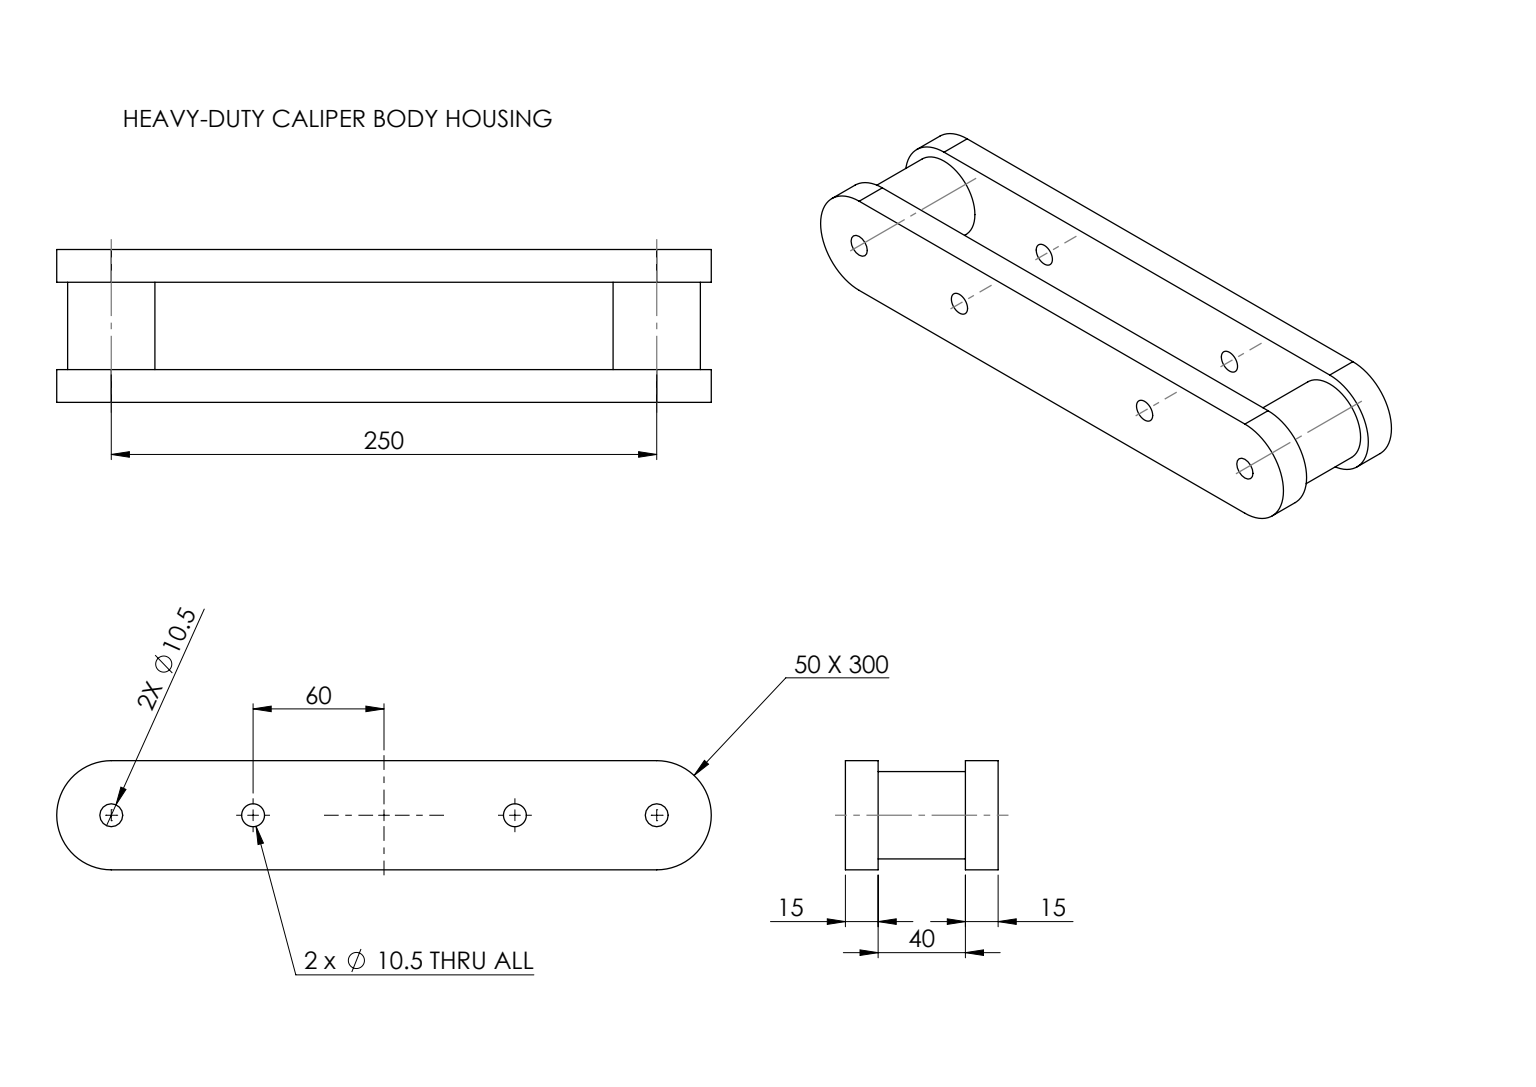
ISO-10303-21;
HEADER;
FILE_DESCRIPTION (('STEP AP214'),
    '1' );
FILE_NAME ('Heavy-Duty Caliper Body Housing.step',
    '2026-10-08T07:58:12',
    ( '' ),
    ( '' ),
    'SwSTEP 2.0',
    'SolidWorks 2026',
    '' );
FILE_SCHEMA (( 'AUTOMOTIVE_DESIGN' ));
ENDSEC;

DATA;
#32=DIRECTION ( 'NONE',  ( -0.000000000000000000, -0.000000000000000000, -1.000000000000000000 ) ) ;
#36=EDGE_CURVE ( 'NONE', #1409, #6493, #16652, .T. ) ;
#53=CARTESIAN_POINT ( 'NONE',  ( 124.3127766070272315, 5.250000000000032863, 35.00001199999999812 ) ) ;
#166=CYLINDRICAL_SURFACE ( 'NONE', #13806, 5.249999999999991118 ) ;
#182=AXIS2_PLACEMENT_3D ( 'NONE', #23295, #23628, #33351 ) ;
#218=CARTESIAN_POINT ( 'NONE',  ( 127.6439996469472220, 4.587378538859885779, 35.00001200000000523 ) ) ;
#239=EDGE_LOOP ( 'NONE', ( #2645, #22396, #19117, #16780 ) ) ;
#303=CARTESIAN_POINT ( 'NONE',  ( 120.4126214611401195, -2.643999646947191362, 35.00001199999999812 ) ) ;
#334=( NAMED_UNIT ( * ) PLANE_ANGLE_UNIT ( ) SI_UNIT ( $, .RADIAN. ) );
#365=ORIENTED_EDGE ( 'NONE', *, *, #11822, .F. ) ;
#449=EDGE_LOOP ( 'NONE', ( #2882, #4117, #25704, #19508 ) ) ;
#451=ORIENTED_EDGE ( 'NONE', *, *, #3089, .T. ) ;
#458=DIRECTION ( 'NONE',  ( 0.000000000000000000, 0.000000000000000000, 1.000000000000000000 ) ) ;
#474=CARTESIAN_POINT ( 'NONE',  ( 122.3560003530528064, -4.587378538859826271, 35.00001200000000523 ) ) ;
#498=CARTESIAN_POINT ( 'NONE',  ( -105.0000000000000142, 2.449293598294705330E-15, 35.00200000000000244 ) ) ;
#553=CARTESIAN_POINT ( 'NONE',  ( -65.24999999999998579, -6.704941225331758039E-15, -20.00000000000000355 ) ) ;
#676=DIRECTION ( 'NONE',  ( -0.000000000000000000, -0.000000000000000000, -1.000000000000000000 ) ) ;
#709=CARTESIAN_POINT ( 'NONE',  ( -125.0000000000000000, 0.000000000000000000, 35.00000000000000000 ) ) ;
#766=PLANE ( 'NONE',  #3114 ) ;
#791=ADVANCED_FACE ( 'NONE', ( #31825 ), #29110, .T. ) ;
#806=CARTESIAN_POINT ( 'NONE',  ( -130.2500000000000000, 6.429395695523609083E-16, 35.00000599999999906 ) ) ;
#827=EDGE_CURVE ( 'NONE', #18269, #18960, #27386, .T. ) ;
#830=EDGE_LOOP ( 'NONE', ( #26379, #19429, #20513, #9975 ) ) ;
#901=AXIS2_PLACEMENT_3D ( 'NONE', #15694, #7192, #17748 ) ;
#981=AXIS2_PLACEMENT_3D ( 'NONE', #30181, #6671, #17224 ) ;
#995=AXIS2_PLACEMENT_3D ( 'NONE', #7458, #17673, #4722 ) ;
#998=ORIENTED_EDGE ( 'NONE', *, *, #28348, .F. ) ;
#1003=CYLINDRICAL_SURFACE ( 'NONE', #10395, 5.250000000000004441 ) ;
#1032=VERTEX_POINT ( 'NONE', #28244 ) ;
#1037=FACE_OUTER_BOUND ( 'NONE', #7836, .T. ) ;
#1048=DIRECTION ( 'NONE',  ( 0.000000000000000000, 0.000000000000000000, 1.000000000000000000 ) ) ;
#1075=CARTESIAN_POINT ( 'NONE',  ( 65.24999999999998579, 7.347880794884118356E-15, -35.00000000000000000 ) ) ;
#1137=CARTESIAN_POINT ( 'NONE',  ( 125.0000000000000000, 3.061616997868383121E-14, -35.00000000000000000 ) ) ;
#1148=VERTEX_POINT ( 'NONE', #15462 ) ;
#1203=DIRECTION ( 'NONE',  ( 1.000000000000000000, 0.000000000000000000, 0.000000000000000000 ) ) ;
#1273=FACE_OUTER_BOUND ( 'NONE', #22824, .T. ) ;
#1312=CARTESIAN_POINT ( 'NONE',  ( -119.7500000000000000, -6.429395695523609083E-16, 35.00000599999999906 ) ) ;
#1340=DIRECTION ( 'NONE',  ( 1.000000000000000000, 0.000000000000000000, 0.000000000000000000 ) ) ;
#1384=EDGE_CURVE ( 'NONE', #5506, #3951, #5563, .T. ) ;
#1398=ORIENTED_EDGE ( 'NONE', *, *, #9346, .T. ) ;
#1409=VERTEX_POINT ( 'NONE', #4355 ) ;
#1453=VERTEX_POINT ( 'NONE', #9126 ) ;
#1473=CARTESIAN_POINT ( 'NONE',  ( -123.6258236071137446, -5.113356552508658837, 35.00001199999999102 ) ) ;
#1515=DIRECTION ( 'NONE',  ( -0.000000000000000000, -0.000000000000000000, 1.000000000000000000 ) ) ;
#1557=CARTESIAN_POINT ( 'NONE',  ( -54.75000000000000711, -7.347880794884118356E-15, 35.00000000000000000 ) ) ;
#1616=CARTESIAN_POINT ( 'NONE',  ( 105.0000000000000142, 3.061616997868383121E-14, 20.00000000000000000 ) ) ;
#1638=CARTESIAN_POINT ( 'NONE',  ( -127.6439996469471936, -4.587378538859854693, 35.00001199999999812 ) ) ;
#1678=DIRECTION ( 'NONE',  ( 1.000000000000000000, 0.000000000000000000, 0.000000000000000000 ) ) ;
#1712=DIRECTION ( 'NONE',  ( 1.000000000000000000, 0.000000000000000000, 0.000000000000000000 ) ) ;
#1757=CARTESIAN_POINT ( 'NONE',  ( -119.7500000000000000, 0.000000000000000000, -35.00000000000000000 ) ) ;
#1793=ADVANCED_FACE ( 'NONE', ( #14914 ), #12360, .F. ) ;
#1818=EDGE_CURVE ( 'NONE', #1032, #16785, #2654, .T. ) ;
#1850=CARTESIAN_POINT ( 'NONE',  ( -125.0000000000000000, 0.000000000000000000, -35.00000000000000000 ) ) ;
#1937=CARTESIAN_POINT ( 'NONE',  ( 145.0000000000000000, 3.306546357697854049E-14, 20.00000000000000000 ) ) ;
#1976=CARTESIAN_POINT ( 'NONE',  ( -119.7500000000000000, 0.6872233929727673551, 35.00001200000000523 ) ) ;
#2010=AXIS2_PLACEMENT_3D ( 'NONE', #12064, #22453, #9339 ) ;
#2025=LINE ( 'NONE', #7138, #23818 ) ;
#2027=EDGE_CURVE ( 'NONE', #20133, #13309, #33132, .T. ) ;
#2063=EDGE_CURVE ( 'NONE', #1148, #11257, #24961, .T. ) ;
#2069=DIRECTION ( 'NONE',  ( -0.000000000000000000, -0.000000000000000000, 1.000000000000000000 ) ) ;
#2080=DIRECTION ( 'NONE',  ( -0.000000000000000000, -0.000000000000000000, 1.000000000000000000 ) ) ;
#2096=CARTESIAN_POINT ( 'NONE',  ( -125.0000000000000000, 0.000000000000000000, -35.00000000000000000 ) ) ;
#2101=CARTESIAN_POINT ( 'NONE',  ( 128.2263702798682630, 4.198250922590480272, 35.00001199999999102 ) ) ;
#2106=DIRECTION ( 'NONE',  ( 1.000000000000000000, 0.000000000000000000, 0.000000000000000000 ) ) ;
#2119=VECTOR ( 'NONE', #32, 1000.000000000000000 ) ;
#2139=ORIENTED_EDGE ( 'NONE', *, *, #26065, .T. ) ;
#2141=ORIENTED_EDGE ( 'NONE', *, *, #2063, .T. ) ;
#2154=CARTESIAN_POINT ( 'NONE',  ( -130.1133565525086908, 1.374176392886221842, 35.00001199999999812 ) ) ;
#2177=CARTESIAN_POINT ( 'NONE',  ( -125.0000000000000000, 0.000000000000000000, 20.00000000000000000 ) ) ;
#2195=DIRECTION ( 'NONE',  ( 1.000000000000000000, 1.804112415015879625E-16, 0.000000000000000000 ) ) ;
#2212=EDGE_LOOP ( 'NONE', ( #10140, #20740 ) ) ;
#2221=VERTEX_POINT ( 'NONE', #12106 ) ;
#2319=CARTESIAN_POINT ( 'NONE',  ( -124.3127766070272457, 5.250000000000003553, 35.00001199999999812 ) ) ;
#2367=CYLINDRICAL_SURFACE ( 'NONE', #23840, 5.250000000000004441 ) ;
#2396=ORIENTED_EDGE ( 'NONE', *, *, #14305, .T. ) ;
#2404=AXIS2_PLACEMENT_3D ( 'NONE', #8872, #11941, #4266 ) ;
#2522=FACE_OUTER_BOUND ( 'NONE', #239, .T. ) ;
#2555=CIRCLE ( 'NONE', #3607, 5.249999999999991118 ) ;
#2602=ORIENTED_EDGE ( 'NONE', *, *, #5442, .T. ) ;
#2645=ORIENTED_EDGE ( 'NONE', *, *, #30971, .F. ) ;
#2646=CIRCLE ( 'NONE', #4824, 24.99999999999999289 ) ;
#2654=LINE ( 'NONE', #10493, #13003 ) ;
#2691=DIRECTION ( 'NONE',  ( 0.000000000000000000, 0.000000000000000000, 1.000000000000000000 ) ) ;
#2709=CARTESIAN_POINT ( 'NONE',  ( -150.0000000000000000, 0.000000000000000000, 35.00000000000000000 ) ) ;
#2713=DIRECTION ( 'NONE',  ( -0.000000000000000000, -0.000000000000000000, 1.000000000000000000 ) ) ;
#2745=SURFACE_STYLE_USAGE ( .BOTH. , #15337 ) ;
#2766=ORIENTED_EDGE ( 'NONE', *, *, #20533, .F. ) ;
#2819=CYLINDRICAL_SURFACE ( 'NONE', #22161, 5.249999999999991118 ) ;
#2828=CARTESIAN_POINT ( 'NONE',  ( 60.00000000000000000, 7.347880794884118356E-15, 20.00000000000000000 ) ) ;
#2846=ADVANCED_FACE ( 'NONE', ( #16494 ), #1003, .F. ) ;
#2847=UNCERTAINTY_MEASURE_WITH_UNIT (LENGTH_MEASURE( 1.000000000000000082E-05 ), #3926, 'distance_accuracy_value', 'NONE');
#2866=CARTESIAN_POINT ( 'NONE',  ( 60.00000000000000000, 7.347880794884118356E-15, 35.00000000000000000 ) ) ;
#2882=ORIENTED_EDGE ( 'NONE', *, *, #26989, .F. ) ;
#2884=CARTESIAN_POINT ( 'NONE',  ( 125.0000000000000000, 4.592425496802574367E-14, -35.00000000000000000 ) ) ;
#2885=CARTESIAN_POINT ( 'NONE',  ( -125.0000000000000000, 25.00000000000000000, 35.00000000000000000 ) ) ;
#2889=ORIENTED_EDGE ( 'NONE', *, *, #31198, .F. ) ;
#2900=AXIS2_PLACEMENT_3D ( 'NONE', #17674, #5401, #30974 ) ;
#2946=EDGE_CURVE ( 'NONE', #18729, #27759, #24526, .T. ) ;
#3042=ORIENTED_EDGE ( 'NONE', *, *, #9485, .F. ) ;
#3089=EDGE_CURVE ( 'NONE', #29773, #2221, #25646, .T. ) ;
#3114=AXIS2_PLACEMENT_3D ( 'NONE', #16595, #21713, #11668 ) ;
#3126=EDGE_CURVE ( 'NONE', #11257, #1148, #10416, .T. ) ;
#3132=PRODUCT_DEFINITION ( 'UNKNOWN', '', #13711, #29523 ) ;
#3197=VECTOR ( 'NONE', #28640, 1000.000000000000000 ) ;
#3212=DIRECTION ( 'NONE',  ( 1.000000000000000000, 1.804112415015879378E-16, 0.000000000000000000 ) ) ;
#3274=ORIENTED_EDGE ( 'NONE', *, *, #5485, .F. ) ;
#3275=CARTESIAN_POINT ( 'NONE',  ( -125.0000000000000000, 0.000000000000000000, -35.00000000000000000 ) ) ;
#3281=CARTESIAN_POINT ( 'NONE',  ( 54.74999999999999289, 7.990820364436481039E-15, 35.00000000000000000 ) ) ;
#3309=AXIS2_PLACEMENT_3D ( 'NONE', #30637, #14619, #6614 ) ;
#3322=CARTESIAN_POINT ( 'NONE',  ( -65.24999999999998579, -6.704941225331758828E-15, 35.00000000000000000 ) ) ;
#3378=CARTESIAN_POINT ( 'NONE',  ( 65.25000000000000000, 7.347880794884118356E-15, 35.00000000000000000 ) ) ;
#3391=CARTESIAN_POINT ( 'NONE',  ( 145.0000000000000000, 3.306546357697854049E-14, 35.00200000000000244 ) ) ;
#3423=LINE ( 'NONE', #13985, #15074 ) ;
#3456=ORIENTED_EDGE ( 'NONE', *, *, #16863, .T. ) ;
#3500=FACE_OUTER_BOUND ( 'NONE', #21099, .T. ) ;
#3517=CARTESIAN_POINT ( 'NONE',  ( 128.2263702798683198, -4.198250922590419876, 35.00001199999999812 ) ) ;
#3542=ADVANCED_FACE ( 'NONE', ( #22038 ), #24430, .T. ) ;
#3547=EDGE_LOOP ( 'NONE', ( #31464, #2889, #14472, #25548 ) ) ;
#3578=CARTESIAN_POINT ( 'NONE',  ( 125.0000000000000000, 25.00000000000004619, -35.00000000000000000 ) ) ;
#3607=AXIS2_PLACEMENT_3D ( 'NONE', #8665, #19390, #14111 ) ;
#3613=DIRECTION ( 'NONE',  ( -1.000000000000000000, 0.000000000000000000, 0.000000000000000000 ) ) ;
#3663=CARTESIAN_POINT ( 'NONE',  ( -125.0000000000000000, -25.00000000000000000, 35.00000000000000000 ) ) ;
#3669=VERTEX_POINT ( 'NONE', #15964 ) ;
#3682=DIRECTION ( 'NONE',  ( 1.000000000000000000, 0.000000000000000000, 0.000000000000000000 ) ) ;
#3693=VECTOR ( 'NONE', #4424, 1000.000000000000000 ) ;
#3781=CARTESIAN_POINT ( 'NONE',  ( 60.00000000000000000, 7.347880794884118356E-15, 35.00000000000000000 ) ) ;
#3784=EDGE_CURVE ( 'NONE', #4076, #18960, #30535, .T. ) ;
#3793=EDGE_LOOP ( 'NONE', ( #21926, #28936 ) ) ;
#3822=DIRECTION ( 'NONE',  ( 0.000000000000000000, 0.000000000000000000, 1.000000000000000000 ) ) ;
#3832=VERTEX_POINT ( 'NONE', #1757 ) ;
#3841=CARTESIAN_POINT ( 'NONE',  ( -125.0000000000000000, 0.000000000000000000, 20.00000000000000000 ) ) ;
#3868=AXIS2_PLACEMENT_3D ( 'NONE', #14876, #17772, #6874 ) ;
#3926=( LENGTH_UNIT ( ) NAMED_UNIT ( * ) SI_UNIT ( .MILLI., .METRE. ) );
#3932=CARTESIAN_POINT ( 'NONE',  ( -60.00000000000000000, -7.347880794884118356E-15, 35.00000000000000000 ) ) ;
#3936=CARTESIAN_POINT ( 'NONE',  ( -60.00000000000000000, -7.347880794884118356E-15, 35.00000000000000000 ) ) ;
#3951=VERTEX_POINT ( 'NONE', #12156 ) ;
#3974=CARTESIAN_POINT ( 'NONE',  ( -125.0000000000000000, 0.000000000000000000, 20.00000000000000000 ) ) ;
#4005=ORIENTED_EDGE ( 'NONE', *, *, #26473, .T. ) ;
#4025=CARTESIAN_POINT ( 'NONE',  ( -54.75000000000000711, -7.347880794884118356E-15, 20.00000000000000000 ) ) ;
#4055=DIRECTION ( 'NONE',  ( -0.000000000000000000, -0.000000000000000000, -1.000000000000000000 ) ) ;
#4066=CARTESIAN_POINT ( 'NONE',  ( -125.0000000000000000, -25.00000000000000000, -35.00000000000000000 ) ) ;
#4076=VERTEX_POINT ( 'NONE', #18116 ) ;
#4081=EDGE_LOOP ( 'NONE', ( #30312, #10229, #3042, #32399 ) ) ;
#4086=ORIENTED_EDGE ( 'NONE', *, *, #19258, .F. ) ;
#4110=LINE ( 'NONE', #6677, #4867 ) ;
#4115=CARTESIAN_POINT ( 'NONE',  ( 125.0000000000000000, 25.00000000000004619, -20.00000000000000000 ) ) ;
#4117=ORIENTED_EDGE ( 'NONE', *, *, #11444, .T. ) ;
#4165=AXIS2_PLACEMENT_3D ( 'NONE', #14276, #16662, #24676 ) ;
#4230=FACE_BOUND ( 'NONE', #27225, .T. ) ;
#4236=VECTOR ( 'NONE', #32723, 1000.000000000000000 ) ;
#4247=EDGE_LOOP ( 'NONE', ( #2141, #30712 ) ) ;
#4266=DIRECTION ( 'NONE',  ( 1.000000000000000000, 0.000000000000000000, 0.000000000000000000 ) ) ;
#4294=ORIENTED_EDGE ( 'NONE', *, *, #5442, .F. ) ;
#4315=FACE_BOUND ( 'NONE', #4247, .T. ) ;
#4355=CARTESIAN_POINT ( 'NONE',  ( -145.0000000000000000, 0.000000000000000000, -20.00000000000000000 ) ) ;
#4392=CARTESIAN_POINT ( 'NONE',  ( 125.0000000000000000, -24.99999999999995737, -35.00000000000000000 ) ) ;
#4416=VERTEX_POINT ( 'NONE', #29845 ) ;
#4424=DIRECTION ( 'NONE',  ( -1.000000000000000000, -1.804112415015879378E-16, -0.000000000000000000 ) ) ;
#4515=ORIENTED_EDGE ( 'NONE', *, *, #26989, .T. ) ;
#4531=CARTESIAN_POINT ( 'NONE',  ( -119.7500000000000000, -6.429395695523609083E-16, 35.00000599999999906 ) ) ;
#4554=ORIENTED_EDGE ( 'NONE', *, *, #12518, .T. ) ;
#4560=FACE_BOUND ( 'NONE', #31244, .T. ) ;
#4570=CARTESIAN_POINT ( 'NONE',  ( 125.0000000000000000, 3.061616997868383121E-14, 20.00000000000000000 ) ) ;
#4578=FACE_OUTER_BOUND ( 'NONE', #30029, .T. ) ;
#4585=CARTESIAN_POINT ( 'NONE',  ( 125.0000000000000000, -24.99999999999995737, 35.00000000000000000 ) ) ;
#4619=CARTESIAN_POINT ( 'NONE',  ( 125.0000000000000000, 4.592425496802574367E-14, 35.00000000000000000 ) ) ;
#4626=DIRECTION ( 'NONE',  ( 1.000000000000000000, 0.000000000000000000, 0.000000000000000000 ) ) ;
#4681=ORIENTED_EDGE ( 'NONE', *, *, #6446, .F. ) ;
#4697=CARTESIAN_POINT ( 'NONE',  ( -129.5873785388598662, 2.643999646947224669, 35.00001200000000523 ) ) ;
#4718=ORIENTED_EDGE ( 'NONE', *, *, #16395, .F. ) ;
#4722=DIRECTION ( 'NONE',  ( 1.000000000000000000, 0.000000000000000000, 0.000000000000000000 ) ) ;
#4824=AXIS2_PLACEMENT_3D ( 'NONE', #2884, #31989, #11215 ) ;
#4842=ORIENTED_EDGE ( 'NONE', *, *, #7670, .T. ) ;
#4867=VECTOR ( 'NONE', #24740, 1000.000000000000000 ) ;
#4871=CARTESIAN_POINT ( 'NONE',  ( -120.8017490774095393, 3.226370279868306046, 35.00001199999999812 ) ) ;
#4971=DIRECTION ( 'NONE',  ( -0.000000000000000000, -0.000000000000000000, 1.000000000000000000 ) ) ;
#5009=CYLINDRICAL_SURFACE ( 'NONE', #24085, 24.99999999999999289 ) ;
#5109=VECTOR ( 'NONE', #24322, 1000.000000000000000 ) ;
#5154=CARTESIAN_POINT ( 'NONE',  ( 130.2499999999999716, 2.997323040913146538E-14, 35.00000599999999906 ) ) ;
#5182=EDGE_CURVE ( 'NONE', #27759, #29773, #16673, .T. ) ;
#5205=DIRECTION ( 'NONE',  ( -1.000000000000000000, 0.000000000000000000, 0.000000000000000000 ) ) ;
#5229=DIRECTION ( 'NONE',  ( 1.000000000000000000, 0.000000000000000000, 0.000000000000000000 ) ) ;
#5234=EDGE_CURVE ( 'NONE', #3669, #1409, #24012, .T. ) ;
#5293=AXIS2_PLACEMENT_3D ( 'NONE', #22069, #32452, #9121 ) ;
#5296=LINE ( 'NONE', #23852, #3197 ) ;
#5309=AXIS2_PLACEMENT_3D ( 'NONE', #3663, #21890, #14562 ) ;
#5366=AXIS2_PLACEMENT_3D ( 'NONE', #1137, #17143, #30261 ) ;
#5401=DIRECTION ( 'NONE',  ( 0.000000000000000000, 0.000000000000000000, 1.000000000000000000 ) ) ;
#5404=EDGE_CURVE ( 'NONE', #16947, #12552, #15663, .T. ) ;
#5409=LINE ( 'NONE', #15794, #15409 ) ;
#5436=EDGE_CURVE ( 'NONE', #18269, #18184, #27091, .T. ) ;
#5442=EDGE_CURVE ( 'NONE', #20128, #3832, #10270, .T. ) ;
#5467=LINE ( 'NONE', #7867, #2119 ) ;
#5485=EDGE_CURVE ( 'NONE', #5632, #16267, #29820, .T. ) ;
#5501=VERTEX_POINT ( 'NONE', #4066 ) ;
#5506=VERTEX_POINT ( 'NONE', #25353 ) ;
#5563=LINE ( 'NONE', #22581, #27625 ) ;
#5580=CARTESIAN_POINT ( 'NONE',  ( -130.2500000000000000, -0.6872233929727670221, 35.00001200000000523 ) ) ;
#5589=VECTOR ( 'NONE', #19251, 1000.000000000000000 ) ;
#5632=VERTEX_POINT ( 'NONE', #23085 ) ;
#5644=CARTESIAN_POINT ( 'NONE',  ( 65.25000000000000000, 7.347880794884118356E-15, 35.00000000000000000 ) ) ;
#5665=DIRECTION ( 'NONE',  ( -0.000000000000000000, -0.000000000000000000, -1.000000000000000000 ) ) ;
#5682=AXIS2_PLACEMENT_3D ( 'NONE', #22806, #18204, #33196 ) ;
#5714=ORIENTED_EDGE ( 'NONE', *, *, #5436, .T. ) ;
#5759=CARTESIAN_POINT ( 'NONE',  ( 125.0000000000000000, 4.592425496802574367E-14, 35.00000000000000000 ) ) ;
#5928=DIRECTION ( 'NONE',  ( -1.000000000000000000, 0.000000000000000000, 0.000000000000000000 ) ) ;
#5996=DIRECTION ( 'NONE',  ( 1.000000000000000000, 0.000000000000000000, 0.000000000000000000 ) ) ;
#6018=( LENGTH_UNIT ( ) NAMED_UNIT ( * ) SI_UNIT ( .MILLI., .METRE. ) );
#6131=DIRECTION ( 'NONE',  ( -0.000000000000000000, -0.000000000000000000, 1.000000000000000000 ) ) ;
#6188=AXIS2_PLACEMENT_3D ( 'NONE', #19777, #9222, #6662 ) ;
#6206=DIRECTION ( 'NONE',  ( 1.000000000000000000, 0.000000000000000000, 0.000000000000000000 ) ) ;
#6211=VECTOR ( 'NONE', #27403, 1000.000000000000000 ) ;
#6238=DIRECTION ( 'NONE',  ( 0.000000000000000000, 0.000000000000000000, 1.000000000000000000 ) ) ;
#6317=DIRECTION ( 'NONE',  ( -0.000000000000000000, -0.000000000000000000, 1.000000000000000000 ) ) ;
#6350=CARTESIAN_POINT ( 'NONE',  ( -119.7500000000000000, -6.429395695523609083E-16, 35.00000599999999906 ) ) ;
#6381=VERTEX_POINT ( 'NONE', #31146 ) ;
#6389=ORIENTED_EDGE ( 'NONE', *, *, #25989, .F. ) ;
#6414=FACE_OUTER_BOUND ( 'NONE', #3547, .T. ) ;
#6415=CARTESIAN_POINT ( 'NONE',  ( 129.1982509225904039, -3.226370279868275404, 35.00001200000000523 ) ) ;
#6419=CARTESIAN_POINT ( 'NONE',  ( -129.1982509225904892, -3.226370279868305602, 35.00001200000000523 ) ) ;
#6446=EDGE_CURVE ( 'NONE', #15275, #4416, #11049, .T. ) ;
#6451=DIRECTION ( 'NONE',  ( -0.000000000000000000, -0.000000000000000000, 1.000000000000000000 ) ) ;
#6493=VERTEX_POINT ( 'NONE', #19357 ) ;
#6568=DIRECTION ( 'NONE',  ( 1.000000000000000000, 0.000000000000000000, 0.000000000000000000 ) ) ;
#6583=CARTESIAN_POINT ( 'NONE',  ( -129.5873785388598662, -2.643999646947223336, 35.00001199999999812 ) ) ;
#6614=DIRECTION ( 'NONE',  ( -1.000000000000000000, 0.000000000000000000, 0.000000000000000000 ) ) ;
#6662=DIRECTION ( 'NONE',  ( -1.000000000000000000, 0.000000000000000000, 0.000000000000000000 ) ) ;
#6671=DIRECTION ( 'NONE',  ( 0.000000000000000000, 0.000000000000000000, 1.000000000000000000 ) ) ;
#6677=CARTESIAN_POINT ( 'NONE',  ( 125.0000000000000000, -24.99999999999995737, -35.00000000000000000 ) ) ;
#6684=FACE_OUTER_BOUND ( 'NONE', #29573, .T. ) ;
#6733=ORIENTED_EDGE ( 'NONE', *, *, #16415, .T. ) ;
#6745=( GEOMETRIC_REPRESENTATION_CONTEXT ( 3 ) GLOBAL_UNCERTAINTY_ASSIGNED_CONTEXT ( ( #2847 ) ) GLOBAL_UNIT_ASSIGNED_CONTEXT ( ( #3926, #32542, #30168 ) ) REPRESENTATION_CONTEXT ( 'NONE', 'WORKASPACE' ) );
#6792=FACE_BOUND ( 'NONE', #21223, .T. ) ;
#6856=VERTEX_POINT ( 'NONE', #33155 ) ;
#6859=DIRECTION ( 'NONE',  ( 1.000000000000000000, 0.000000000000000000, 0.000000000000000000 ) ) ;
#6870=PLANE ( 'NONE',  #12389 ) ;
#6874=DIRECTION ( 'NONE',  ( -1.000000000000000000, 0.000000000000000000, 0.000000000000000000 ) ) ;
#6896=ADVANCED_FACE ( 'NONE', ( #10158 ), #7772, .T. ) ;
#6916=CIRCLE ( 'NONE', #2010, 5.250000000000004441 ) ;
#6968=DIRECTION ( 'NONE',  ( 1.000000000000000000, 0.000000000000000000, 0.000000000000000000 ) ) ;
#6989=LINE ( 'NONE', #24870, #3693 ) ;
#7097=DIRECTION ( 'NONE',  ( -1.000000000000000000, 0.000000000000000000, 0.000000000000000000 ) ) ;
#7118=DIRECTION ( 'NONE',  ( 1.000000000000000000, 0.000000000000000000, 0.000000000000000000 ) ) ;
#7135=FACE_BOUND ( 'NONE', #2212, .T. ) ;
#7136=CARTESIAN_POINT ( 'NONE',  ( 125.0000000000000000, 3.061616997868383121E-14, -35.00000000000000000 ) ) ;
#7138=CARTESIAN_POINT ( 'NONE',  ( -130.2500000000000000, 6.429395695523609083E-16, -35.00000000000000000 ) ) ;
#7147=EDGE_LOOP ( 'NONE', ( #19157, #8854, #31862, #26570, #3456 ) ) ;
#7151=CARTESIAN_POINT ( 'NONE',  ( 65.25000000000000000, 7.347880794884118356E-15, 20.00000000000000000 ) ) ;
#7192=DIRECTION ( 'NONE',  ( -0.000000000000000000, -0.000000000000000000, 1.000000000000000000 ) ) ;
#7255=CARTESIAN_POINT ( 'NONE',  ( -150.0000000000000000, 0.000000000000000000, 20.00000000000000000 ) ) ;
#7265=CARTESIAN_POINT ( 'NONE',  ( -127.6439996469472788, 4.587378538859859134, 35.00001200000001234 ) ) ;
#7276=CIRCLE ( 'NONE', #8915, 24.99999999999999289 ) ;
#7279=CARTESIAN_POINT ( 'NONE',  ( -125.0000000000000000, 25.00000000000000000, -20.00000000000000000 ) ) ;
#7290=ORIENTED_EDGE ( 'NONE', *, *, #1384, .F. ) ;
#7330=DIRECTION ( 'NONE',  ( -0.000000000000000000, -0.000000000000000000, -1.000000000000000000 ) ) ;
#7358=CARTESIAN_POINT ( 'NONE',  ( 60.00000000000000000, 7.347880794884118356E-15, 35.00000000000000000 ) ) ;
#7375=DIRECTION ( 'NONE',  ( 0.000000000000000000, 0.000000000000000000, 1.000000000000000000 ) ) ;
#7382=CARTESIAN_POINT ( 'NONE',  ( 119.8866434474913660, 1.374176392886252707, 35.00001199999999812 ) ) ;
#7408=DIRECTION ( 'NONE',  ( 0.000000000000000000, 0.000000000000000000, 1.000000000000000000 ) ) ;
#7411=ORIENTED_EDGE ( 'NONE', *, *, #1384, .T. ) ;
#7458=CARTESIAN_POINT ( 'NONE',  ( -125.0000000000000000, 0.000000000000000000, -35.00000000000000000 ) ) ;
#7465=CYLINDRICAL_SURFACE ( 'NONE', #14006, 24.99999999999999289 ) ;
#7476=CARTESIAN_POINT ( 'NONE',  ( 123.6258236071138015, -5.113356552508631303, 35.00001199999999812 ) ) ;
#7503=CARTESIAN_POINT ( 'NONE',  ( -150.0000000000000000, 0.000000000000000000, -35.00000000000000000 ) ) ;
#7583=CARTESIAN_POINT ( 'NONE',  ( -54.75000000000000711, -7.347880794884118356E-15, -35.00000000000000000 ) ) ;
#7594=CIRCLE ( 'NONE', #22111, 19.99999999999998934 ) ;
#7608=CARTESIAN_POINT ( 'NONE',  ( -125.0000000000000000, 0.000000000000000000, -35.00000000000000000 ) ) ;
#7663=EDGE_CURVE ( 'NONE', #5501, #10405, #33627, .T. ) ;
#7668=VERTEX_POINT ( 'NONE', #10306 ) ;
#7670=EDGE_CURVE ( 'NONE', #23420, #10127, #20682, .T. ) ;
#7690=CARTESIAN_POINT ( 'NONE',  ( 119.7500000000000000, 3.125910954823619074E-14, -35.00000000000000000 ) ) ;
#7720=CARTESIAN_POINT ( 'NONE',  ( 123.6258236071137731, 5.113356552508689923, 35.00001199999999812 ) ) ;
#7727=EDGE_CURVE ( 'NONE', #6493, #1409, #24418, .T. ) ;
#7763=CARTESIAN_POINT ( 'NONE',  ( -125.0000000000000000, 25.00000000000000000, 35.00000000000000000 ) ) ;
#7772=CYLINDRICAL_SURFACE ( 'NONE', #22768, 24.99999999999999289 ) ;
#7796=FACE_BOUND ( 'NONE', #12090, .T. ) ;
#7836=EDGE_LOOP ( 'NONE', ( #20686, #24416, #10641, #2396 ) ) ;
#7865=EDGE_CURVE ( 'NONE', #6856, #5501, #25002, .T. ) ;
#7867=CARTESIAN_POINT ( 'NONE',  ( 105.0000000000000142, 3.061616997868383121E-14, 35.00200000000000244 ) ) ;
#7888=ORIENTED_EDGE ( 'NONE', *, *, #5436, .F. ) ;
#7933=DIRECTION ( 'NONE',  ( 1.000000000000000000, 1.804112415015879378E-16, 0.000000000000000000 ) ) ;
#7937=FACE_OUTER_BOUND ( 'NONE', #9195, .T. ) ;
#7959=EDGE_LOOP ( 'NONE', ( #16994, #25241 ) ) ;
#7972=DIRECTION ( 'NONE',  ( -1.000000000000000000, 0.000000000000000000, 0.000000000000000000 ) ) ;
#7997=LINE ( 'NONE', #13756, #10185 ) ;
#8006=DIRECTION ( 'NONE',  ( 1.000000000000000000, 0.000000000000000000, 0.000000000000000000 ) ) ;
#8031=AXIS2_PLACEMENT_3D ( 'NONE', #19112, #11123, #29848 ) ;
#8036=ORIENTED_EDGE ( 'NONE', *, *, #9090, .T. ) ;
#8068=AXIS2_PLACEMENT_3D ( 'NONE', #7136, #29801, #25182 ) ;
#8088=EDGE_CURVE ( 'NONE', #10405, #5632, #4110, .T. ) ;
#8151=CARTESIAN_POINT ( 'NONE',  ( 121.7736297201317370, -4.198250922590419876, 35.00001200000000523 ) ) ;
#8156=ADVANCED_FACE ( 'NONE', ( #22171 ), #21834, .F. ) ;
#8198=CYLINDRICAL_SURFACE ( 'NONE', #33357, 5.249999999999991118 ) ;
#8210=CYLINDRICAL_SURFACE ( 'NONE', #24907, 5.250000000000004441 ) ;
#8216=EDGE_LOOP ( 'NONE', ( #3274, #18721, #19449, #27462 ) ) ;
#8245=VERTEX_POINT ( 'NONE', #30186 ) ;
#8283=EDGE_LOOP ( 'NONE', ( #2139, #7290, #365, #32066 ) ) ;
#8302=DIRECTION ( 'NONE',  ( -1.000000000000000000, 0.000000000000000000, 0.000000000000000000 ) ) ;
#8317=AXIS2_PLACEMENT_3D ( 'NONE', #29351, #13341, #3613 ) ;
#8338=EDGE_LOOP ( 'NONE', ( #19377, #29267 ) ) ;
#8340=CIRCLE ( 'NONE', #11066, 5.249999999999997335 ) ;
#8375=DIRECTION ( 'NONE',  ( -0.000000000000000000, -0.000000000000000000, 1.000000000000000000 ) ) ;
#8544=DIRECTION ( 'NONE',  ( -0.000000000000000000, -0.000000000000000000, 1.000000000000000000 ) ) ;
#8548=CIRCLE ( 'NONE', #5293, 24.99999999999999289 ) ;
#8606=DIRECTION ( 'NONE',  ( -0.000000000000000000, -0.000000000000000000, 1.000000000000000000 ) ) ;
#8665=CARTESIAN_POINT ( 'NONE',  ( -60.00000000000000000, -7.347880794884118356E-15, -35.00000000000000000 ) ) ;
#8761=AXIS2_PLACEMENT_3D ( 'NONE', #14378, #10866, #8302 ) ;
#8810=ORIENTED_EDGE ( 'NONE', *, *, #23076, .F. ) ;
#8816=DIRECTION ( 'NONE',  ( -0.000000000000000000, -0.000000000000000000, -1.000000000000000000 ) ) ;
#8821=EDGE_LOOP ( 'NONE', ( #21758, #8810, #9214, #19710 ) ) ;
#8831=PRODUCT_CONTEXT ( 'NONE', #15940, 'mechanical' ) ;
#8839=B_SPLINE_CURVE_WITH_KNOTS ( 'NONE', 3,
 ( #806, #5580, #14419, #6583, #6419, #14928, #1638, #24812, #22255, #30437, #1473, #11868, #32642, #32470, #32808, #9305, #27863, #1312 ),
 .UNSPECIFIED., .F., .F.,
 ( 4, 2, 2, 2, 2, 2, 2, 2, 4 ),
 ( 0.5000000000000000000, 0.5625000000000006661, 0.6250000000000012212, 0.6875000000000018874, 0.7500000000000024425, 0.8125000000000018874, 0.8750000000000013323, 0.9375000000000006661, 1.000000000000000000 ),
 .UNSPECIFIED. ) ;
#8854=ORIENTED_EDGE ( 'NONE', *, *, #22897, .T. ) ;
#8871=CARTESIAN_POINT ( 'NONE',  ( -125.0000000000000000, 0.000000000000000000, 35.00000000000000000 ) ) ;
#8872=CARTESIAN_POINT ( 'NONE',  ( 0.000000000000000000, 0.000000000000000000, 0.000000000000000000 ) ) ;
#8889=ORIENTED_EDGE ( 'NONE', *, *, #14591, .F. ) ;
#8890=DIRECTION ( 'NONE',  ( 1.000000000000000000, 0.000000000000000000, 0.000000000000000000 ) ) ;
#8906=LINE ( 'NONE', #13852, #12159 ) ;
#8915=AXIS2_PLACEMENT_3D ( 'NONE', #4619, #9898, #1712 ) ;
#9088=AXIS2_PLACEMENT_3D ( 'NONE', #10941, #21317, #1203 ) ;
#9090=EDGE_CURVE ( 'NONE', #23420, #20358, #22693, .T. ) ;
#9114=PLANE ( 'NONE',  #5309 ) ;
#9121=DIRECTION ( 'NONE',  ( 1.000000000000000000, 0.000000000000000000, 0.000000000000000000 ) ) ;
#9126=CARTESIAN_POINT ( 'NONE',  ( -65.24999999999998579, -6.704941225331758039E-15, 20.00000000000000000 ) ) ;
#9184=FACE_BOUND ( 'NONE', #11465, .T. ) ;
#9185=CARTESIAN_POINT ( 'NONE',  ( 125.0000000000000000, 4.592425496802574367E-14, -20.00000000000000000 ) ) ;
#9195=EDGE_LOOP ( 'NONE', ( #31710, #14568, #11514, #12815 ) ) ;
#9214=ORIENTED_EDGE ( 'NONE', *, *, #29256, .T. ) ;
#9218=AXIS2_PLACEMENT_3D ( 'NONE', #32562, #22340, #8890 ) ;
#9222=DIRECTION ( 'NONE',  ( -0.000000000000000000, -0.000000000000000000, -1.000000000000000000 ) ) ;
#9239=DIRECTION ( 'NONE',  ( -0.000000000000000000, -0.000000000000000000, -1.000000000000000000 ) ) ;
#9263=DIRECTION ( 'NONE',  ( 1.000000000000000000, 0.000000000000000000, 0.000000000000000000 ) ) ;
#9293=ADVANCED_FACE ( 'NONE', ( #1273 ), #766, .F. ) ;
#9305=CARTESIAN_POINT ( 'NONE',  ( -119.8866434474913518, -1.374176392886225617, 35.00001199999999812 ) ) ;
#9339=DIRECTION ( 'NONE',  ( 1.000000000000000000, 0.000000000000000000, 0.000000000000000000 ) ) ;
#9346=EDGE_CURVE ( 'NONE', #13309, #31209, #28146, .T. ) ;
#9378=SURFACE_STYLE_FILL_AREA ( #9544 ) ;
#9485=EDGE_CURVE ( 'NONE', #7668, #27493, #24874, .T. ) ;
#9504=DIRECTION ( 'NONE',  ( -1.000000000000000000, 0.000000000000000000, 0.000000000000000000 ) ) ;
#9517=EDGE_CURVE ( 'NONE', #20358, #22384, #3423, .T. ) ;
#9533=EDGE_LOOP ( 'NONE', ( #7888, #9952, #13263, #31460 ) ) ;
#9544=FILL_AREA_STYLE ('',( #22662 ) ) ;
#9578=DIRECTION ( 'NONE',  ( -0.000000000000000000, -0.000000000000000000, 1.000000000000000000 ) ) ;
#9670=ORIENTED_EDGE ( 'NONE', *, *, #31256, .T. ) ;
#9671=DIRECTION ( 'NONE',  ( -1.000000000000000000, 0.000000000000000000, 0.000000000000000000 ) ) ;
#9691=AXIS2_PLACEMENT_3D ( 'NONE', #7358, #2069, #4626 ) ;
#9732=AXIS2_PLACEMENT_3D ( 'NONE', #13338, #26613, #14003 ) ;
#9802=EDGE_LOOP ( 'NONE', ( #4718, #4086, #17440, #4554 ) ) ;
#9844=FACE_BOUND ( 'NONE', #20821, .T. ) ;
#9876=CARTESIAN_POINT ( 'NONE',  ( 125.0000000000000000, -24.99999999999995737, 35.00000000000000000 ) ) ;
#9878=ORIENTED_EDGE ( 'NONE', *, *, #16395, .T. ) ;
#9898=DIRECTION ( 'NONE',  ( 0.000000000000000000, 0.000000000000000000, 1.000000000000000000 ) ) ;
#9927=AXIS2_PLACEMENT_3D ( 'NONE', #16626, #19190, #3682 ) ;
#9935=CARTESIAN_POINT ( 'NONE',  ( 130.1133565525086908, 1.374176392886252485, 35.00001199999999812 ) ) ;
#9952=ORIENTED_EDGE ( 'NONE', *, *, #827, .T. ) ;
#9973=ORIENTED_EDGE ( 'NONE', *, *, #7727, .F. ) ;
#9975=ORIENTED_EDGE ( 'NONE', *, *, #36, .T. ) ;
#10022=FACE_BOUND ( 'NONE', #30836, .T. ) ;
#10078=( NAMED_UNIT ( * ) SI_UNIT ( $, .STERADIAN. ) SOLID_ANGLE_UNIT ( ) );
#10127=VERTEX_POINT ( 'NONE', #3378 ) ;
#10131=FACE_OUTER_BOUND ( 'NONE', #14524, .T. ) ;
#10140=ORIENTED_EDGE ( 'NONE', *, *, #19258, .T. ) ;
#10158=FACE_OUTER_BOUND ( 'NONE', #4081, .T. ) ;
#10185=VECTOR ( 'NONE', #28774, 1000.000000000000000 ) ;
#10209=CARTESIAN_POINT ( 'NONE',  ( -125.0000000000000000, 25.00000000000000000, -35.00000000000000000 ) ) ;
#10229=ORIENTED_EDGE ( 'NONE', *, *, #25342, .T. ) ;
#10232=DIRECTION ( 'NONE',  ( -0.000000000000000000, -0.000000000000000000, 1.000000000000000000 ) ) ;
#10270=CIRCLE ( 'NONE', #32528, 5.250000000000004441 ) ;
#10293=PRODUCT_DEFINITION_SHAPE ( 'NONE', 'NONE',  #3132 ) ;
#10296=AXIS2_PLACEMENT_3D ( 'NONE', #29837, #27270, #14325 ) ;
#10306=CARTESIAN_POINT ( 'NONE',  ( -125.0000000000000000, 25.00000000000000000, -20.00000000000000000 ) ) ;
#10314=VECTOR ( 'NONE', #10468, 1000.000000000000000 ) ;
#10352=ORIENTED_EDGE ( 'NONE', *, *, #9517, .F. ) ;
#10377=FACE_OUTER_BOUND ( 'NONE', #30484, .T. ) ;
#10395=AXIS2_PLACEMENT_3D ( 'NONE', #29788, #31831, #21278 ) ;
#10398=ADVANCED_FACE ( 'NONE', ( #22616 ), #14444, .T. ) ;
#10405=VERTEX_POINT ( 'NONE', #4392 ) ;
#10416=CIRCLE ( 'NONE', #27268, 5.249999999999991118 ) ;
#10468=DIRECTION ( 'NONE',  ( 1.000000000000000000, 1.804112415015879378E-16, 0.000000000000000000 ) ) ;
#10493=CARTESIAN_POINT ( 'NONE',  ( -125.0000000000000000, -25.00000000000000000, 20.00000000000000000 ) ) ;
#10503=DIRECTION ( 'NONE',  ( -0.000000000000000000, -0.000000000000000000, 1.000000000000000000 ) ) ;
#10507=CARTESIAN_POINT ( 'NONE',  ( 145.0000000000000000, 3.306546357697854049E-14, -20.00000000000000355 ) ) ;
#10527=FACE_OUTER_BOUND ( 'NONE', #11847, .T. ) ;
#10565=CARTESIAN_POINT ( 'NONE',  ( -60.00000000000000000, -7.347880794884118356E-15, 35.00000000000000000 ) ) ;
#10610=ADVANCED_FACE ( 'NONE', ( #20232 ), #7465, .T. ) ;
#10615=CARTESIAN_POINT ( 'NONE',  ( 126.3741763928862269, 5.113356552508691699, 35.00001199999999102 ) ) ;
#10641=ORIENTED_EDGE ( 'NONE', *, *, #23480, .T. ) ;
#10721=AXIS2_PLACEMENT_3D ( 'NONE', #3841, #17300, #6568 ) ;
#10726=ADVANCED_FACE ( 'NONE', ( #2522 ), #20741, .T. ) ;
#10751=DIRECTION ( 'NONE',  ( -0.000000000000000000, -0.000000000000000000, 1.000000000000000000 ) ) ;
#10866=DIRECTION ( 'NONE',  ( -0.000000000000000000, -0.000000000000000000, -1.000000000000000000 ) ) ;
#10871=CARTESIAN_POINT ( 'NONE',  ( 126.3741763928862554, -5.113356552508631303, 35.00001200000001234 ) ) ;
#10941=CARTESIAN_POINT ( 'NONE',  ( -125.0000000000000000, 0.000000000000000000, -20.00000000000000000 ) ) ;
#11049=B_SPLINE_CURVE_WITH_KNOTS ( 'NONE', 3,
 ( #15801, #23475, #23643, #303, #31484, #8151, #474, #7476, #24135, #27195, #10871, #21412, #3517, #6415, #29250, #19192, #14243, #11192 ),
 .UNSPECIFIED., .F., .F.,
 ( 4, 2, 2, 2, 2, 2, 2, 2, 4 ),
 ( 0.5000000000000000000, 0.5624999999999993339, 0.6249999999999986677, 0.6874999999999981126, 0.7499999999999974465, 0.8124999999999980016, 0.8749999999999986677, 0.9374999999999993339, 1.000000000000000000 ),
 .UNSPECIFIED. ) ;
#11066=AXIS2_PLACEMENT_3D ( 'NONE', #3932, #6317, #14330 ) ;
#11123=DIRECTION ( 'NONE',  ( -0.000000000000000000, -0.000000000000000000, 1.000000000000000000 ) ) ;
#11183=EDGE_CURVE ( 'NONE', #12431, #6856, #20868, .T. ) ;
#11184=DIRECTION ( 'NONE',  ( -1.000000000000000000, 0.000000000000000000, 0.000000000000000000 ) ) ;
#11192=CARTESIAN_POINT ( 'NONE',  ( 130.2499999999999716, 2.997323040913146538E-14, 35.00000599999999906 ) ) ;
#11215=DIRECTION ( 'NONE',  ( 1.000000000000000000, 0.000000000000000000, 0.000000000000000000 ) ) ;
#11257=VERTEX_POINT ( 'NONE', #553 ) ;
#11260=VERTEX_POINT ( 'NONE', #31068 ) ;
#11299=ORIENTED_EDGE ( 'NONE', *, *, #28462, .T. ) ;
#11361=FACE_BOUND ( 'NONE', #16389, .T. ) ;
#11444=EDGE_CURVE ( 'NONE', #12552, #15275, #16543, .T. ) ;
#11465=EDGE_LOOP ( 'NONE', ( #8036, #21352 ) ) ;
#11473=EDGE_CURVE ( 'NONE', #11260, #20519, #8340, .T. ) ;
#11514=ORIENTED_EDGE ( 'NONE', *, *, #2063, .F. ) ;
#11531=CARTESIAN_POINT ( 'NONE',  ( 125.0000000000000000, 3.061616997868383121E-14, -20.00000000000000355 ) ) ;
#11549=LINE ( 'NONE', #24497, #26885 ) ;
#11591=ORIENTED_EDGE ( 'NONE', *, *, #24948, .T. ) ;
#11648=AXIS2_PLACEMENT_3D ( 'NONE', #3936, #22846, #11951 ) ;
#11652=DIRECTION ( 'NONE',  ( 0.000000000000000000, 0.000000000000000000, -1.000000000000000000 ) ) ;
#11666=ADVANCED_FACE ( 'NONE', ( #33232 ), #15001, .T. ) ;
#11668=DIRECTION ( 'NONE',  ( -1.000000000000000000, -1.804112415015879625E-16, -0.000000000000000000 ) ) ;
#11762=ORIENTED_EDGE ( 'NONE', *, *, #36, .F. ) ;
#11813=FACE_BOUND ( 'NONE', #19756, .T. ) ;
#11822=EDGE_CURVE ( 'NONE', #32913, #5506, #7276, .T. ) ;
#11847=EDGE_LOOP ( 'NONE', ( #17875, #14273, #25885, #27730, #23547 ) ) ;
#11868=CARTESIAN_POINT ( 'NONE',  ( -122.3560003530527780, -4.587378538859857358, 35.00001199999999812 ) ) ;
#11883=MANIFOLD_SOLID_BREP ( 'M10 Clearance Hole1', #26993 ) ;
#11895=AXIS2_PLACEMENT_3D ( 'NONE', #15951, #458, #16284 ) ;
#11941=DIRECTION ( 'NONE',  ( 0.000000000000000000, 0.000000000000000000, 1.000000000000000000 ) ) ;
#11951=DIRECTION ( 'NONE',  ( 1.000000000000000000, 0.000000000000000000, 0.000000000000000000 ) ) ;
#11963=ORIENTED_EDGE ( 'NONE', *, *, #24948, .F. ) ;
#12010=ORIENTED_EDGE ( 'NONE', *, *, #1818, .T. ) ;
#12064=CARTESIAN_POINT ( 'NONE',  ( 125.0000000000000000, 3.061616997868383121E-14, -35.00000000000000000 ) ) ;
#12090=EDGE_LOOP ( 'NONE', ( #31404, #4515 ) ) ;
#12106=CARTESIAN_POINT ( 'NONE',  ( 105.0000000000000142, 3.061616997868383121E-14, -20.00000000000000355 ) ) ;
#12153=VECTOR ( 'NONE', #8544, 1000.000000000000000 ) ;
#12156=CARTESIAN_POINT ( 'NONE',  ( 125.0000000000000000, 25.00000000000004619, 20.00000000000000000 ) ) ;
#12159=VECTOR ( 'NONE', #16738, 1000.000000000000000 ) ;
#12181=ORIENTED_EDGE ( 'NONE', *, *, #27992, .T. ) ;
#12270=SHAPE_REPRESENTATION_RELATIONSHIP ( 'NONE' , 'NONE' ,  #13706, #31568 ) ;
#12297=CARTESIAN_POINT ( 'NONE',  ( 125.0000000000000000, 3.061616997868383121E-14, 35.00200000000000244 ) ) ;
#12351=ORIENTED_EDGE ( 'NONE', *, *, #28082, .T. ) ;
#12355=AXIS2_PLACEMENT_3D ( 'NONE', #2828, #3822, #6206 ) ;
#12360=PLANE ( 'NONE',  #26578 ) ;
#12367=CARTESIAN_POINT ( 'NONE',  ( -121.7736297201317086, 4.198250922590448297, 35.00001199999999812 ) ) ;
#12389=AXIS2_PLACEMENT_3D ( 'NONE', #16749, #11652, #14700 ) ;
#12403=AXIS2_PLACEMENT_3D ( 'NONE', #9185, #16843, #14965 ) ;
#12425=EDGE_CURVE ( 'NONE', #13309, #33143, #29166, .T. ) ;
#12431=VERTEX_POINT ( 'NONE', #23887 ) ;
#12442=VECTOR ( 'NONE', #25696, 1000.000000000000000 ) ;
#12488=CARTESIAN_POINT ( 'NONE',  ( 125.6872233929728111, 5.250000000000034639, 35.00001200000001234 ) ) ;
#12494=CARTESIAN_POINT ( 'NONE',  ( -125.0000000000000000, 0.000000000000000000, -35.00000000000000000 ) ) ;
#12518=EDGE_CURVE ( 'NONE', #20519, #11260, #19816, .T. ) ;
#12537=CARTESIAN_POINT ( 'NONE',  ( -130.2499999999999716, 0.6872233929727687984, 35.00001199999999102 ) ) ;
#12552=VERTEX_POINT ( 'NONE', #7690 ) ;
#12612=PRESENTATION_STYLE_ASSIGNMENT (( #2745 ) ) ;
#12666=ORIENTED_EDGE ( 'NONE', *, *, #20956, .F. ) ;
#12815=ORIENTED_EDGE ( 'NONE', *, *, #12896, .F. ) ;
#12871=VECTOR ( 'NONE', #13968, 1000.000000000000000 ) ;
#12896=EDGE_CURVE ( 'NONE', #17833, #1148, #22625, .T. ) ;
#12902=ADVANCED_FACE ( 'NONE', ( #7135, #9184, #4230, #6792, #4578 ), #27236, .F. ) ;
#12906=CARTESIAN_POINT ( 'NONE',  ( -125.0000000000000000, 0.000000000000000000, 35.00200000000000244 ) ) ;
#12977=AXIS2_PLACEMENT_3D ( 'NONE', #22626, #14454, #1678 ) ;
#13003=VECTOR ( 'NONE', #7933, 1000.000000000000000 ) ;
#13017=CARTESIAN_POINT ( 'NONE',  ( -125.0000000000000000, 0.000000000000000000, -35.00000000000000000 ) ) ;
#13045=CARTESIAN_POINT ( 'NONE',  ( 119.7500000000000000, 3.125910954823619074E-14, 35.00000599999999906 ) ) ;
#13130=ADVANCED_FACE ( 'NONE', ( #10377 ), #15477, .F. ) ;
#13132=ADVANCED_FACE ( 'NONE', ( #25868 ), #23145, .F. ) ;
#13202=CARTESIAN_POINT ( 'NONE',  ( -60.00000000000000000, -7.347880794884118356E-15, 35.00000000000000000 ) ) ;
#13252=AXIS2_PLACEMENT_3D ( 'NONE', #30370, #7375, #32917 ) ;
#13263=ORIENTED_EDGE ( 'NONE', *, *, #3784, .F. ) ;
#13267=EDGE_LOOP ( 'NONE', ( #27757, #26458, #15207, #14181 ) ) ;
#13271=VECTOR ( 'NONE', #29340, 1000.000000000000000 ) ;
#13309=VERTEX_POINT ( 'NONE', #2709 ) ;
#13338=CARTESIAN_POINT ( 'NONE',  ( -125.0000000000000000, 0.000000000000000000, -20.00000000000000000 ) ) ;
#13341=DIRECTION ( 'NONE',  ( -0.000000000000000000, -0.000000000000000000, -1.000000000000000000 ) ) ;
#13395=CIRCLE ( 'NONE', #901, 24.99999999999999289 ) ;
#13422=ORIENTED_EDGE ( 'NONE', *, *, #7865, .T. ) ;
#13430=CARTESIAN_POINT ( 'NONE',  ( -54.75000000000000000, -7.347880794884118356E-15, 35.00000000000000000 ) ) ;
#13545=ORIENTED_EDGE ( 'NONE', *, *, #7670, .F. ) ;
#13595=VERTEX_POINT ( 'NONE', #4025 ) ;
#13706=SHAPE_REPRESENTATION ( 'Heavy-Duty Caliper Body Housing', ( #2404 ), #33408 ) ;
#13711=PRODUCT_DEFINITION_FORMATION_WITH_SPECIFIED_SOURCE ( 'ANY', '', #28508, .NOT_KNOWN. ) ;
#13720=UNCERTAINTY_MEASURE_WITH_UNIT (LENGTH_MEASURE( 1.000000000000000082E-05 ), #17903, 'distance_accuracy_value', 'NONE');
#13756=CARTESIAN_POINT ( 'NONE',  ( 130.2500000000000000, 3.061616997868383121E-14, -35.00000000000000000 ) ) ;
#13806=AXIS2_PLACEMENT_3D ( 'NONE', #10565, #31336, #8006 ) ;
#13852=CARTESIAN_POINT ( 'NONE',  ( -125.0000000000000000, -25.00000000000000000, 35.00000000000000000 ) ) ;
#13877=EDGE_CURVE ( 'NONE', #21298, #32783, #17298, .T. ) ;
#13952=CARTESIAN_POINT ( 'NONE',  ( -145.0000000000000000, 0.000000000000000000, 35.00200000000000244 ) ) ;
#13954=DIRECTION ( 'NONE',  ( -0.000000000000000000, -0.000000000000000000, 1.000000000000000000 ) ) ;
#13968=DIRECTION ( 'NONE',  ( -0.000000000000000000, -0.000000000000000000, 1.000000000000000000 ) ) ;
#13985=CARTESIAN_POINT ( 'NONE',  ( 54.75000000000000000, 7.990820364436479461E-15, 35.00000000000000000 ) ) ;
#14003=DIRECTION ( 'NONE',  ( 1.000000000000000000, 0.000000000000000000, 0.000000000000000000 ) ) ;
#14006=AXIS2_PLACEMENT_3D ( 'NONE', #33521, #31308, #7972 ) ;
#14070=VECTOR ( 'NONE', #25952, 1000.000000000000000 ) ;
#14111=DIRECTION ( 'NONE',  ( 1.000000000000000000, 0.000000000000000000, 0.000000000000000000 ) ) ;
#14181=ORIENTED_EDGE ( 'NONE', *, *, #25989, .T. ) ;
#14243=CARTESIAN_POINT ( 'NONE',  ( 130.2500000000000284, -0.6872233929727383783, 35.00001200000001234 ) ) ;
#14273=ORIENTED_EDGE ( 'NONE', *, *, #29256, .F. ) ;
#14276=CARTESIAN_POINT ( 'NONE',  ( 60.00000000000000000, 7.347880794884118356E-15, -20.00000000000000355 ) ) ;
#14305=EDGE_CURVE ( 'NONE', #4416, #15275, #25875, .T. ) ;
#14319=AXIS2_PLACEMENT_3D ( 'NONE', #2096, #9578, #6859 ) ;
#14325=DIRECTION ( 'NONE',  ( -1.000000000000000000, 0.000000000000000000, 0.000000000000000000 ) ) ;
#14330=DIRECTION ( 'NONE',  ( 1.000000000000000000, 0.000000000000000000, 0.000000000000000000 ) ) ;
#14378=CARTESIAN_POINT ( 'NONE',  ( -125.0000000000000000, 0.000000000000000000, 35.00200000000000244 ) ) ;
#14419=CARTESIAN_POINT ( 'NONE',  ( -130.1133565525086908, -1.374176392886221620, 35.00001199999999812 ) ) ;
#14444=CYLINDRICAL_SURFACE ( 'NONE', #21085, 24.99999999999999289 ) ;
#14454=DIRECTION ( 'NONE',  ( -0.000000000000000000, -0.000000000000000000, 1.000000000000000000 ) ) ;
#14472=ORIENTED_EDGE ( 'NONE', *, *, #12896, .T. ) ;
#14493=AXIS2_PLACEMENT_3D ( 'NONE', #22390, #7408, #20353 ) ;
#14524=EDGE_LOOP ( 'NONE', ( #25857, #13422, #15369, #32731 ) ) ;
#14562=DIRECTION ( 'NONE',  ( -1.000000000000000000, -1.804112415015879625E-16, 0.000000000000000000 ) ) ;
#14568=ORIENTED_EDGE ( 'NONE', *, *, #17275, .T. ) ;
#14586=CARTESIAN_POINT ( 'NONE',  ( -125.0000000000000000, -25.00000000000000000, -20.00000000000000000 ) ) ;
#14591=EDGE_CURVE ( 'NONE', #5506, #20133, #16536, .T. ) ;
#14601=AXIS2_PLACEMENT_3D ( 'NONE', #11531, #24646, #7097 ) ;
#14619=DIRECTION ( 'NONE',  ( -0.000000000000000000, -0.000000000000000000, 1.000000000000000000 ) ) ;
#14700=DIRECTION ( 'NONE',  ( 1.000000000000000000, 0.000000000000000000, 0.000000000000000000 ) ) ;
#14782=ADVANCED_FACE ( 'NONE', ( #19356, #29248, #11361, #23968, #29085 ), #32131, .T. ) ;
#14872=ADVANCED_FACE ( 'NONE', ( #6414 ), #29413, .F. ) ;
#14876=CARTESIAN_POINT ( 'NONE',  ( 60.00000000000000000, 7.347880794884118356E-15, -20.00000000000000355 ) ) ;
#14904=VECTOR ( 'NONE', #28941, 1000.000000000000000 ) ;
#14914=FACE_OUTER_BOUND ( 'NONE', #18832, .T. ) ;
#14928=CARTESIAN_POINT ( 'NONE',  ( -128.2263702798682630, -4.198250922590447409, 35.00001199999999812 ) ) ;
#14965=DIRECTION ( 'NONE',  ( 1.000000000000000000, 0.000000000000000000, 0.000000000000000000 ) ) ;
#15001=CYLINDRICAL_SURFACE ( 'NONE', #6188, 19.99999999999998934 ) ;
#15074=VECTOR ( 'NONE', #19432, 1000.000000000000000 ) ;
#15079=VECTOR ( 'NONE', #7330, 1000.000000000000000 ) ;
#15155=CIRCLE ( 'NONE', #19507, 24.99999999999999289 ) ;
#15207=ORIENTED_EDGE ( 'NONE', *, *, #30439, .T. ) ;
#15271=LINE ( 'NONE', #7279, #5589 ) ;
#15275=VERTEX_POINT ( 'NONE', #13045 ) ;
#15337=SURFACE_SIDE_STYLE ('',( #26075 ) ) ;
#15369=ORIENTED_EDGE ( 'NONE', *, *, #31855, .T. ) ;
#15377=CARTESIAN_POINT ( 'NONE',  ( 120.4126214611401480, 2.643999646947254423, 35.00001199999999812 ) ) ;
#15406=ORIENTED_EDGE ( 'NONE', *, *, #9090, .F. ) ;
#15409=VECTOR ( 'NONE', #26185, 1000.000000000000000 ) ;
#15462=CARTESIAN_POINT ( 'NONE',  ( -54.75000000000000711, -7.347880794884118356E-15, -20.00000000000000355 ) ) ;
#15477=CYLINDRICAL_SURFACE ( 'NONE', #5682, 5.250000000000004441 ) ;
#15542=CARTESIAN_POINT ( 'NONE',  ( 130.2500000000000284, 0.6872233929727983304, 35.00001200000000523 ) ) ;
#15654=VECTOR ( 'NONE', #5665, 1000.000000000000000 ) ;
#15660=LINE ( 'NONE', #31015, #14904 ) ;
#15663=CIRCLE ( 'NONE', #8068, 5.250000000000004441 ) ;
#15694=CARTESIAN_POINT ( 'NONE',  ( -125.0000000000000000, 0.000000000000000000, -20.00000000000000000 ) ) ;
#15781=ADVANCED_FACE ( 'NONE', ( #10131 ), #5009, .T. ) ;
#15794=CARTESIAN_POINT ( 'NONE',  ( -125.0000000000000000, -25.00000000000000000, -35.00000000000000000 ) ) ;
#15801=CARTESIAN_POINT ( 'NONE',  ( 119.7500000000000000, 3.125910954823619074E-14, 35.00000599999999906 ) ) ;
#15831=ORIENTED_EDGE ( 'NONE', *, *, #31256, .F. ) ;
#15860=ADVANCED_FACE ( 'NONE', ( #20848 ), #18957, .T. ) ;
#15940=APPLICATION_CONTEXT ( 'automotive_design' ) ;
#15951=CARTESIAN_POINT ( 'NONE',  ( 125.0000000000000000, 4.592425496802574367E-14, 20.00000000000000000 ) ) ;
#15964=CARTESIAN_POINT ( 'NONE',  ( -145.0000000000000000, 0.000000000000000000, 20.00000000000000000 ) ) ;
#16004=FILL_AREA_STYLE_COLOUR ( '', #18699 ) ;
#16041=DIRECTION ( 'NONE',  ( 1.000000000000000000, 0.000000000000000000, 0.000000000000000000 ) ) ;
#16059=DIRECTION ( 'NONE',  ( -0.000000000000000000, -0.000000000000000000, 1.000000000000000000 ) ) ;
#16152=DIRECTION ( 'NONE',  ( -0.000000000000000000, -0.000000000000000000, -1.000000000000000000 ) ) ;
#16267=VERTEX_POINT ( 'NONE', #4115 ) ;
#16278=ORIENTED_EDGE ( 'NONE', *, *, #827, .F. ) ;
#16284=DIRECTION ( 'NONE',  ( 1.000000000000000000, 0.000000000000000000, 0.000000000000000000 ) ) ;
#16316=ORIENTED_EDGE ( 'NONE', *, *, #2946, .T. ) ;
#16389=EDGE_LOOP ( 'NONE', ( #31215, #4681 ) ) ;
#16395=EDGE_CURVE ( 'NONE', #1453, #11260, #25917, .T. ) ;
#16415=EDGE_CURVE ( 'NONE', #18184, #18269, #31217, .T. ) ;
#16494=FACE_OUTER_BOUND ( 'NONE', #33285, .T. ) ;
#16521=LINE ( 'NONE', #3578, #12871 ) ;
#16536=LINE ( 'NONE', #18933, #32768 ) ;
#16543=LINE ( 'NONE', #18939, #12153 ) ;
#16595=CARTESIAN_POINT ( 'NONE',  ( -125.0000000000000000, -25.00000000000000000, -35.00000000000000000 ) ) ;
#16607=EDGE_LOOP ( 'NONE', ( #21877, #1398, #31375, #18430, #21309 ) ) ;
#16626=CARTESIAN_POINT ( 'NONE',  ( -60.00000000000000000, -7.347880794884118356E-15, 35.00000000000000000 ) ) ;
#16652=CIRCLE ( 'NONE', #14493, 19.99999999999998934 ) ;
#16662=DIRECTION ( 'NONE',  ( 0.000000000000000000, 0.000000000000000000, -1.000000000000000000 ) ) ;
#16673=LINE ( 'NONE', #3391, #27756 ) ;
#16675=CARTESIAN_POINT ( 'NONE',  ( -125.0000000000000000, 25.00000000000000000, 20.00000000000000000 ) ) ;
#16713=CIRCLE ( 'NONE', #8031, 5.249999999999991118 ) ;
#16738=DIRECTION ( 'NONE',  ( 1.000000000000000000, 1.804112415015879378E-16, 0.000000000000000000 ) ) ;
#16741=FACE_OUTER_BOUND ( 'NONE', #33681, .T. ) ;
#16744=ORIENTED_EDGE ( 'NONE', *, *, #30419, .T. ) ;
#16749=CARTESIAN_POINT ( 'NONE',  ( -125.0000000000000000, 0.000000000000000000, -20.00000000000000000 ) ) ;
#16780=ORIENTED_EDGE ( 'NONE', *, *, #5234, .F. ) ;
#16785=VERTEX_POINT ( 'NONE', #29140 ) ;
#16843=DIRECTION ( 'NONE',  ( -0.000000000000000000, -0.000000000000000000, 1.000000000000000000 ) ) ;
#16855=EDGE_LOOP ( 'NONE', ( #23199, #21987 ) ) ;
#16863=EDGE_CURVE ( 'NONE', #16267, #7668, #15271, .T. ) ;
#16908=CYLINDRICAL_SURFACE ( 'NONE', #14319, 5.250000000000004441 ) ;
#16947=VERTEX_POINT ( 'NONE', #21972 ) ;
#16989=CYLINDRICAL_SURFACE ( 'NONE', #28540, 5.250000000000004441 ) ;
#16994=ORIENTED_EDGE ( 'NONE', *, *, #13877, .F. ) ;
#16999=DIRECTION ( 'NONE',  ( 0.000000000000000000, 0.000000000000000000, -1.000000000000000000 ) ) ;
#17058=LINE ( 'NONE', #1557, #4236 ) ;
#17073=DIRECTION ( 'NONE',  ( -1.000000000000000000, 0.000000000000000000, 0.000000000000000000 ) ) ;
#17098=FACE_OUTER_BOUND ( 'NONE', #7147, .T. ) ;
#17143=DIRECTION ( 'NONE',  ( -0.000000000000000000, -0.000000000000000000, 1.000000000000000000 ) ) ;
#17159=ORIENTED_EDGE ( 'NONE', *, *, #26065, .F. ) ;
#17224=DIRECTION ( 'NONE',  ( 1.000000000000000000, 0.000000000000000000, 0.000000000000000000 ) ) ;
#17275=EDGE_CURVE ( 'NONE', #8245, #11257, #31936, .T. ) ;
#17298=B_SPLINE_CURVE_WITH_KNOTS ( 'NONE', 3,
 ( #4531, #1976, #28036, #25652, #4871, #12367, #22763, #33156, #2319, #20200, #30600, #7265, #25480, #17648, #4697, #2154, #12537, #22927 ),
 .UNSPECIFIED., .F., .F.,
 ( 4, 2, 2, 2, 2, 2, 2, 2, 4 ),
 ( 0.000000000000000000, 0.06249999999999940326, 0.1249999999999987788, 0.1874999999999981681, 0.2499999999999975298, 0.3124999999999981681, 0.3749999999999987788, 0.4374999999999994449, 0.5000000000000000000 ),
 .UNSPECIFIED. ) ;
#17300=DIRECTION ( 'NONE',  ( 0.000000000000000000, 0.000000000000000000, 1.000000000000000000 ) ) ;
#17328=ORIENTED_EDGE ( 'NONE', *, *, #26552, .F. ) ;
#17440=ORIENTED_EDGE ( 'NONE', *, *, #28348, .T. ) ;
#17531=AXIS2_PLACEMENT_3D ( 'NONE', #18696, #6238, #21410 ) ;
#17648=CARTESIAN_POINT ( 'NONE',  ( -129.1982509225904607, 3.226370279868306490, 35.00001200000000523 ) ) ;
#17673=DIRECTION ( 'NONE',  ( 0.000000000000000000, 0.000000000000000000, -1.000000000000000000 ) ) ;
#17674=CARTESIAN_POINT ( 'NONE',  ( -60.00000000000000000, -7.347880794884118356E-15, 20.00000000000000000 ) ) ;
#17748=DIRECTION ( 'NONE',  ( 1.000000000000000000, 0.000000000000000000, 0.000000000000000000 ) ) ;
#17761=CARTESIAN_POINT ( 'NONE',  ( 119.7500000000000000, 3.125910954823619074E-14, 35.00000599999999906 ) ) ;
#17768=DIRECTION ( 'NONE',  ( 1.000000000000000000, 0.000000000000000000, 0.000000000000000000 ) ) ;
#17772=DIRECTION ( 'NONE',  ( 0.000000000000000000, 0.000000000000000000, -1.000000000000000000 ) ) ;
#17783=DIRECTION ( 'NONE',  ( -0.000000000000000000, -0.000000000000000000, 1.000000000000000000 ) ) ;
#17808=DIRECTION ( 'NONE',  ( 1.804112415015879625E-16, -1.000000000000000000, 0.000000000000000000 ) ) ;
#17833=VERTEX_POINT ( 'NONE', #7583 ) ;
#17875=ORIENTED_EDGE ( 'NONE', *, *, #11183, .F. ) ;
#17903=( LENGTH_UNIT ( ) NAMED_UNIT ( * ) SI_UNIT ( .MILLI., .METRE. ) );
#17944=CARTESIAN_POINT ( 'NONE',  ( 119.7499999999999858, 0.6872233929727994406, 35.00001200000000523 ) ) ;
#18046=LINE ( 'NONE', #9876, #15079 ) ;
#18091=DIRECTION ( 'NONE',  ( 1.804112415015879625E-16, -1.000000000000000000, 0.000000000000000000 ) ) ;
#18116=CARTESIAN_POINT ( 'NONE',  ( 65.25000000000000000, 7.347880794884118356E-15, -20.00000000000000355 ) ) ;
#18150=CIRCLE ( 'NONE', #13252, 5.249999999999991118 ) ;
#18184=VERTEX_POINT ( 'NONE', #1075 ) ;
#18204=DIRECTION ( 'NONE',  ( -0.000000000000000000, -0.000000000000000000, 1.000000000000000000 ) ) ;
#18255=CARTESIAN_POINT ( 'NONE',  ( -65.24999999999998579, -6.704941225331758828E-15, 35.00000000000000000 ) ) ;
#18269=VERTEX_POINT ( 'NONE', #22691 ) ;
#18372=AXIS2_PLACEMENT_3D ( 'NONE', #12906, #27697, #11184 ) ;
#18389=CARTESIAN_POINT ( 'NONE',  ( 54.75000000000000000, 7.990820364436479461E-15, 20.00000000000000000 ) ) ;
#18430=ORIENTED_EDGE ( 'NONE', *, *, #11822, .T. ) ;
#18440=CARTESIAN_POINT ( 'NONE',  ( 129.5873785388598662, 2.643999646947254867, 35.00001199999999812 ) ) ;
#18670=ORIENTED_EDGE ( 'NONE', *, *, #5182, .T. ) ;
#18678=EDGE_LOOP ( 'NONE', ( #29651, #21801, #16744, #26301 ) ) ;
#18696=CARTESIAN_POINT ( 'NONE',  ( -125.0000000000000000, 0.000000000000000000, 35.00000000000000000 ) ) ;
#18699=COLOUR_RGB ( '', 0.66274510, 0.83137255, 0.94901961) ;
#18721=ORIENTED_EDGE ( 'NONE', *, *, #8088, .F. ) ;
#18729=VERTEX_POINT ( 'NONE', #1616 ) ;
#18773=DIRECTION ( 'NONE',  ( 0.000000000000000000, 0.000000000000000000, 1.000000000000000000 ) ) ;
#18832=EDGE_LOOP ( 'NONE', ( #11591, #26990, #8889, #7411 ) ) ;
#18933=CARTESIAN_POINT ( 'NONE',  ( -125.0000000000000000, 25.00000000000000000, 35.00000000000000000 ) ) ;
#18939=CARTESIAN_POINT ( 'NONE',  ( 119.7500000000000000, 3.125910954823619074E-14, -35.00000000000000000 ) ) ;
#18957=CYLINDRICAL_SURFACE ( 'NONE', #8317, 24.99999999999999289 ) ;
#18960=VERTEX_POINT ( 'NONE', #21021 ) ;
#18979=EDGE_CURVE ( 'NONE', #31209, #32913, #8906, .T. ) ;
#18998=ORIENTED_EDGE ( 'NONE', *, *, #30971, .T. ) ;
#19112=CARTESIAN_POINT ( 'NONE',  ( -60.00000000000000000, -7.347880794884118356E-15, -35.00000000000000000 ) ) ;
#19117=ORIENTED_EDGE ( 'NONE', *, *, #7727, .T. ) ;
#19157=ORIENTED_EDGE ( 'NONE', *, *, #9485, .T. ) ;
#19190=DIRECTION ( 'NONE',  ( -0.000000000000000000, -0.000000000000000000, 1.000000000000000000 ) ) ;
#19192=CARTESIAN_POINT ( 'NONE',  ( 130.1133565525086624, -1.374176392886194975, 35.00001200000001234 ) ) ;
#19243=FACE_OUTER_BOUND ( 'NONE', #30841, .T. ) ;
#19251=DIRECTION ( 'NONE',  ( -1.000000000000000000, -1.804112415015879378E-16, 0.000000000000000000 ) ) ;
#19258=EDGE_CURVE ( 'NONE', #13595, #1453, #18150, .T. ) ;
#19259=CARTESIAN_POINT ( 'NONE',  ( 125.0000000000000000, 3.061616997868383121E-14, -35.00000000000000000 ) ) ;
#19270=DIRECTION ( 'NONE',  ( 1.000000000000000000, 0.000000000000000000, 0.000000000000000000 ) ) ;
#19356=FACE_BOUND ( 'NONE', #16855, .T. ) ;
#19357=CARTESIAN_POINT ( 'NONE',  ( -105.0000000000000142, 2.449293598294705330E-15, -20.00000000000000000 ) ) ;
#19377=ORIENTED_EDGE ( 'NONE', *, *, #28462, .F. ) ;
#19381=LINE ( 'NONE', #498, #5109 ) ;
#19390=DIRECTION ( 'NONE',  ( -0.000000000000000000, -0.000000000000000000, 1.000000000000000000 ) ) ;
#19429=ORIENTED_EDGE ( 'NONE', *, *, #26473, .F. ) ;
#19432=DIRECTION ( 'NONE',  ( -0.000000000000000000, -0.000000000000000000, 1.000000000000000000 ) ) ;
#19449=ORIENTED_EDGE ( 'NONE', *, *, #25391, .T. ) ;
#19472=ORIENTED_EDGE ( 'NONE', *, *, #28341, .F. ) ;
#19507=AXIS2_PLACEMENT_3D ( 'NONE', #2177, #2691, #5229 ) ;
#19508=ORIENTED_EDGE ( 'NONE', *, *, #23480, .F. ) ;
#19559=CARTESIAN_POINT ( 'NONE',  ( 54.75000000000000000, 7.990820364436479461E-15, 35.00000000000000000 ) ) ;
#19630=ORIENTED_EDGE ( 'NONE', *, *, #9517, .T. ) ;
#19639=ORIENTED_EDGE ( 'NONE', *, *, #20177, .F. ) ;
#19678=ORIENTED_EDGE ( 'NONE', *, *, #12425, .T. ) ;
#19710=ORIENTED_EDGE ( 'NONE', *, *, #28744, .T. ) ;
#19756=EDGE_LOOP ( 'NONE', ( #11762, #9973 ) ) ;
#19770=ORIENTED_EDGE ( 'NONE', *, *, #3784, .T. ) ;
#19777=CARTESIAN_POINT ( 'NONE',  ( 125.0000000000000000, 3.061616997868383121E-14, 35.00200000000000244 ) ) ;
#19816=CIRCLE ( 'NONE', #11648, 5.249999999999997335 ) ;
#20003=CIRCLE ( 'NONE', #31955, 5.250000000000004441 ) ;
#20019=VECTOR ( 'NONE', #6131, 1000.000000000000000 ) ;
#20027=CIRCLE ( 'NONE', #981, 5.250000000000004441 ) ;
#20128=VERTEX_POINT ( 'NONE', #32701 ) ;
#20133=VERTEX_POINT ( 'NONE', #2885 ) ;
#20151=FACE_BOUND ( 'NONE', #3793, .T. ) ;
#20177=EDGE_CURVE ( 'NONE', #3832, #21298, #15660, .T. ) ;
#20200=CARTESIAN_POINT ( 'NONE',  ( -125.6872233929727827, 5.250000000000003553, 35.00001199999999812 ) ) ;
#20232=FACE_OUTER_BOUND ( 'NONE', #22068, .T. ) ;
#20328=MECHANICAL_DESIGN_GEOMETRIC_PRESENTATION_REPRESENTATION('',(#26308),#33393);
#20347=MECHANICAL_DESIGN_GEOMETRIC_PRESENTATION_REPRESENTATION('',(#30690),#6745);
#20353=DIRECTION ( 'NONE',  ( 1.000000000000000000, 0.000000000000000000, 0.000000000000000000 ) ) ;
#20355=ADVANCED_FACE ( 'NONE', ( #23499 ), #166, .F. ) ;
#20358=VERTEX_POINT ( 'NONE', #18389 ) ;
#20375=EDGE_CURVE ( 'NONE', #6381, #6493, #19381, .T. ) ;
#20490=CARTESIAN_POINT ( 'NONE',  ( 129.1982509225904039, 3.226370279868336244, 35.00001199999999102 ) ) ;
#20513=ORIENTED_EDGE ( 'NONE', *, *, #5234, .T. ) ;
#20519=VERTEX_POINT ( 'NONE', #13430 ) ;
#20533=EDGE_CURVE ( 'NONE', #29612, #5632, #11549, .T. ) ;
#20574=EDGE_CURVE ( 'NONE', #27759, #18729, #25810, .T. ) ;
#20594=DIRECTION ( 'NONE',  ( 1.000000000000000000, 0.000000000000000000, 0.000000000000000000 ) ) ;
#20682=LINE ( 'NONE', #31080, #14070 ) ;
#20686=ORIENTED_EDGE ( 'NONE', *, *, #11444, .F. ) ;
#20719=VECTOR ( 'NONE', #21459, 1000.000000000000000 ) ;
#20740=ORIENTED_EDGE ( 'NONE', *, *, #20920, .T. ) ;
#20741=CYLINDRICAL_SURFACE ( 'NONE', #18372, 19.99999999999998934 ) ;
#20764=ADVANCED_FACE ( 'NONE', ( #32492 ), #16989, .F. ) ;
#20821=EDGE_LOOP ( 'NONE', ( #25767, #2602 ) ) ;
#20848=FACE_OUTER_BOUND ( 'NONE', #13267, .T. ) ;
#20868=CIRCLE ( 'NONE', #24653, 24.99999999999999289 ) ;
#20920=EDGE_CURVE ( 'NONE', #1453, #13595, #32820, .T. ) ;
#20939=ORIENTED_EDGE ( 'NONE', *, *, #28938, .T. ) ;
#20943=LINE ( 'NONE', #7503, #32559 ) ;
#20956=EDGE_CURVE ( 'NONE', #20358, #23420, #29015, .T. ) ;
#21021=CARTESIAN_POINT ( 'NONE',  ( 54.75000000000000000, 7.990820364436479461E-15, -20.00000000000000355 ) ) ;
#21085=AXIS2_PLACEMENT_3D ( 'NONE', #25341, #6451, #9671 ) ;
#21099=EDGE_LOOP ( 'NONE', ( #12010, #33558, #25420, #12181 ) ) ;
#21223=EDGE_LOOP ( 'NONE', ( #4005, #18998 ) ) ;
#21231=UNCERTAINTY_MEASURE_WITH_UNIT (LENGTH_MEASURE( 1.000000000000000082E-05 ), #6018, 'distance_accuracy_value', 'NONE');
#21278=DIRECTION ( 'NONE',  ( 1.000000000000000000, 0.000000000000000000, 0.000000000000000000 ) ) ;
#21284=SHAPE_DEFINITION_REPRESENTATION ( #10293, #13706 ) ;
#21298=VERTEX_POINT ( 'NONE', #6350 ) ;
#21309=ORIENTED_EDGE ( 'NONE', *, *, #14591, .T. ) ;
#21317=DIRECTION ( 'NONE',  ( -0.000000000000000000, -0.000000000000000000, 1.000000000000000000 ) ) ;
#21329=ADVANCED_FACE ( 'NONE', ( #16741 ), #16908, .F. ) ;
#21352=ORIENTED_EDGE ( 'NONE', *, *, #20956, .T. ) ;
#21410=DIRECTION ( 'NONE',  ( 1.000000000000000000, 0.000000000000000000, -0.000000000000000000 ) ) ;
#21412=CARTESIAN_POINT ( 'NONE',  ( 127.6439996469472504, -4.587378538859826271, 35.00001200000000523 ) ) ;
#21431=COLOUR_RGB ( '', 0.66274510, 0.83137255, 0.94901961) ;
#21446=ORIENTED_EDGE ( 'NONE', *, *, #28045, .T. ) ;
#21459=DIRECTION ( 'NONE',  ( -0.000000000000000000, -0.000000000000000000, -1.000000000000000000 ) ) ;
#21499=DIRECTION ( 'NONE',  ( 1.000000000000000000, 0.000000000000000000, 0.000000000000000000 ) ) ;
#21713=DIRECTION ( 'NONE',  ( -1.804112415015879625E-16, 1.000000000000000000, 0.000000000000000000 ) ) ;
#21758=ORIENTED_EDGE ( 'NONE', *, *, #16863, .F. ) ;
#21766=CARTESIAN_POINT ( 'NONE',  ( 125.0000000000000000, 3.061616997868383121E-14, 20.00000000000000000 ) ) ;
#21801=ORIENTED_EDGE ( 'NONE', *, *, #20574, .T. ) ;
#21834=CYLINDRICAL_SURFACE ( 'NONE', #9218, 5.250000000000004441 ) ;
#21877=ORIENTED_EDGE ( 'NONE', *, *, #2027, .T. ) ;
#21890=DIRECTION ( 'NONE',  ( -1.804112415015879625E-16, 1.000000000000000000, 0.000000000000000000 ) ) ;
#21926=ORIENTED_EDGE ( 'NONE', *, *, #29585, .F. ) ;
#21972=CARTESIAN_POINT ( 'NONE',  ( 130.2500000000000000, 3.061616997868383121E-14, -35.00000000000000000 ) ) ;
#21979=ORIENTED_EDGE ( 'NONE', *, *, #13877, .T. ) ;
#21987=ORIENTED_EDGE ( 'NONE', *, *, #11473, .F. ) ;
#22000=AXIS2_PLACEMENT_3D ( 'NONE', #25526, #18091, #2195 ) ;
#22038=FACE_OUTER_BOUND ( 'NONE', #830, .T. ) ;
#22068=EDGE_LOOP ( 'NONE', ( #30490, #19678, #27974, #27248 ) ) ;
#22069=CARTESIAN_POINT ( 'NONE',  ( -125.0000000000000000, 0.000000000000000000, 20.00000000000000000 ) ) ;
#22096=ORIENTED_EDGE ( 'NONE', *, *, #16415, .F. ) ;
#22111=AXIS2_PLACEMENT_3D ( 'NONE', #3974, #27151, #2106 ) ;
#22154=SURFACE_STYLE_USAGE ( .BOTH. , #27269 ) ;
#22161=AXIS2_PLACEMENT_3D ( 'NONE', #13202, #23602, #9263 ) ;
#22171=FACE_OUTER_BOUND ( 'NONE', #32406, .T. ) ;
#22187=VECTOR ( 'NONE', #13954, 1000.000000000000000 ) ;
#22228=CIRCLE ( 'NONE', #11895, 24.99999999999999289 ) ;
#22255=CARTESIAN_POINT ( 'NONE',  ( -125.6872233929727827, -5.250000000000002665, 35.00001199999999812 ) ) ;
#22340=DIRECTION ( 'NONE',  ( -0.000000000000000000, -0.000000000000000000, 1.000000000000000000 ) ) ;
#22346=CYLINDRICAL_SURFACE ( 'NONE', #31903, 19.99999999999998934 ) ;
#22384=VERTEX_POINT ( 'NONE', #3281 ) ;
#22390=CARTESIAN_POINT ( 'NONE',  ( -125.0000000000000000, 0.000000000000000000, -20.00000000000000000 ) ) ;
#22396=ORIENTED_EDGE ( 'NONE', *, *, #20375, .T. ) ;
#22453=DIRECTION ( 'NONE',  ( 0.000000000000000000, 0.000000000000000000, 1.000000000000000000 ) ) ;
#22475=ADVANCED_FACE ( 'NONE', ( #6684 ), #22346, .T. ) ;
#22581=CARTESIAN_POINT ( 'NONE',  ( 125.0000000000000000, 25.00000000000004619, 35.00000000000000000 ) ) ;
#22590=CYLINDRICAL_SURFACE ( 'NONE', #5366, 5.250000000000004441 ) ;
#22616=FACE_OUTER_BOUND ( 'NONE', #8216, .T. ) ;
#22625=LINE ( 'NONE', #33013, #6211 ) ;
#22626=CARTESIAN_POINT ( 'NONE',  ( 60.00000000000000000, 7.347880794884118356E-15, -35.00000000000000000 ) ) ;
#22662=FILL_AREA_STYLE_COLOUR ( '', #21431 ) ;
#22691=CARTESIAN_POINT ( 'NONE',  ( 54.75000000000000711, 7.990820364436479461E-15, -35.00000000000000000 ) ) ;
#22693=CIRCLE ( 'NONE', #12355, 5.250000000000004441 ) ;
#22763=CARTESIAN_POINT ( 'NONE',  ( -122.3560003530527638, 4.587378538859855581, 35.00001199999999812 ) ) ;
#22768=AXIS2_PLACEMENT_3D ( 'NONE', #7608, #10503, #5205 ) ;
#22806=CARTESIAN_POINT ( 'NONE',  ( 60.00000000000000000, 7.347880794884118356E-15, 35.00000000000000000 ) ) ;
#22824=EDGE_LOOP ( 'NONE', ( #2766, #28248, #26143, #31703 ) ) ;
#22846=DIRECTION ( 'NONE',  ( -0.000000000000000000, -0.000000000000000000, 1.000000000000000000 ) ) ;
#22897=EDGE_CURVE ( 'NONE', #27493, #29612, #13395, .T. ) ;
#22927=CARTESIAN_POINT ( 'NONE',  ( -130.2500000000000000, 6.429395695523609083E-16, 35.00000599999999906 ) ) ;
#22953=PLANE ( 'NONE',  #995 ) ;
#23063=EDGE_LOOP ( 'NONE', ( #16278, #22096, #30967, #15831 ) ) ;
#23076=EDGE_CURVE ( 'NONE', #23340, #16267, #16521, .T. ) ;
#23085=CARTESIAN_POINT ( 'NONE',  ( 125.0000000000000000, -24.99999999999995737, -20.00000000000000000 ) ) ;
#23145=PLANE ( 'NONE',  #22000 ) ;
#23161=ORIENTED_EDGE ( 'NONE', *, *, #20920, .F. ) ;
#23199=ORIENTED_EDGE ( 'NONE', *, *, #12518, .F. ) ;
#23295=CARTESIAN_POINT ( 'NONE',  ( 60.00000000000000000, 7.347880794884118356E-15, 20.00000000000000000 ) ) ;
#23340=VERTEX_POINT ( 'NONE', #33384 ) ;
#23420=VERTEX_POINT ( 'NONE', #7151 ) ;
#23461=EDGE_CURVE ( 'NONE', #32913, #16785, #18046, .T. ) ;
#23475=CARTESIAN_POINT ( 'NONE',  ( 119.7500000000000000, -0.6872233929727361579, 35.00001200000000523 ) ) ;
#23480=EDGE_CURVE ( 'NONE', #16947, #4416, #7997, .T. ) ;
#23499=FACE_OUTER_BOUND ( 'NONE', #9802, .T. ) ;
#23547=ORIENTED_EDGE ( 'NONE', *, *, #7865, .F. ) ;
#23602=DIRECTION ( 'NONE',  ( -0.000000000000000000, -0.000000000000000000, 1.000000000000000000 ) ) ;
#23628=DIRECTION ( 'NONE',  ( 0.000000000000000000, 0.000000000000000000, 1.000000000000000000 ) ) ;
#23643=CARTESIAN_POINT ( 'NONE',  ( 119.8866434474913518, -1.374176392886190756, 35.00001199999999102 ) ) ;
#23789=VECTOR ( 'NONE', #25008, 1000.000000000000000 ) ;
#23818=VECTOR ( 'NONE', #1515, 1000.000000000000000 ) ;
#23825=DIRECTION ( 'NONE',  ( 1.000000000000000000, 0.000000000000000000, 0.000000000000000000 ) ) ;
#23840=AXIS2_PLACEMENT_3D ( 'NONE', #2866, #2713, #20594 ) ;
#23846=CARTESIAN_POINT ( 'NONE',  ( -125.0000000000000000, 25.00000000000000000, -35.00000000000000000 ) ) ;
#23850=DIRECTION ( 'NONE',  ( 1.000000000000000000, 0.000000000000000000, 0.000000000000000000 ) ) ;
#23852=CARTESIAN_POINT ( 'NONE',  ( -125.0000000000000000, 25.00000000000000000, 35.00000000000000000 ) ) ;
#23887=CARTESIAN_POINT ( 'NONE',  ( -125.0000000000000000, 25.00000000000000000, -35.00000000000000000 ) ) ;
#23930=ORIENTED_EDGE ( 'NONE', *, *, #28938, .F. ) ;
#23968=FACE_BOUND ( 'NONE', #7959, .T. ) ;
#24012=LINE ( 'NONE', #13952, #20719 ) ;
#24085=AXIS2_PLACEMENT_3D ( 'NONE', #13017, #17783, #28527 ) ;
#24135=CARTESIAN_POINT ( 'NONE',  ( 124.3127766070272457, -5.249999999999974243, 35.00001199999999812 ) ) ;
#24153=ORIENTED_EDGE ( 'NONE', *, *, #20574, .F. ) ;
#24162=ADVANCED_FACE ( 'NONE', ( #3500 ), #9114, .F. ) ;
#24200=APPLICATION_CONTEXT ( 'automotive_design' ) ;
#24322=DIRECTION ( 'NONE',  ( -0.000000000000000000, -0.000000000000000000, -1.000000000000000000 ) ) ;
#24416=ORIENTED_EDGE ( 'NONE', *, *, #5404, .F. ) ;
#24418=CIRCLE ( 'NONE', #9732, 19.99999999999998934 ) ;
#24430=CYLINDRICAL_SURFACE ( 'NONE', #8761, 19.99999999999998934 ) ;
#24497=CARTESIAN_POINT ( 'NONE',  ( -125.0000000000000000, -25.00000000000000000, -20.00000000000000000 ) ) ;
#24526=CIRCLE ( 'NONE', #28878, 19.99999999999998934 ) ;
#24561=DIRECTION ( 'NONE',  ( -0.000000000000000000, -0.000000000000000000, 1.000000000000000000 ) ) ;
#24646=DIRECTION ( 'NONE',  ( -0.000000000000000000, -0.000000000000000000, 1.000000000000000000 ) ) ;
#24653=AXIS2_PLACEMENT_3D ( 'NONE', #12494, #33274, #17768 ) ;
#24676=DIRECTION ( 'NONE',  ( -1.000000000000000000, 0.000000000000000000, 0.000000000000000000 ) ) ;
#24740=DIRECTION ( 'NONE',  ( -0.000000000000000000, -0.000000000000000000, 1.000000000000000000 ) ) ;
#24779=ADVANCED_FACE ( 'NONE', ( #1037 ), #8210, .F. ) ;
#24804=DIRECTION ( 'NONE',  ( -0.000000000000000000, -0.000000000000000000, -1.000000000000000000 ) ) ;
#24812=CARTESIAN_POINT ( 'NONE',  ( -126.3741763928862269, -5.113356552508659725, 35.00001199999999812 ) ) ;
#24870=CARTESIAN_POINT ( 'NONE',  ( -125.0000000000000000, 25.00000000000000000, 20.00000000000000000 ) ) ;
#24874=CIRCLE ( 'NONE', #9088, 24.99999999999999289 ) ;
#24883=( NAMED_UNIT ( * ) PLANE_ANGLE_UNIT ( ) SI_UNIT ( $, .RADIAN. ) );
#24907=AXIS2_PLACEMENT_3D ( 'NONE', #19259, #8375, #31863 ) ;
#24920=EDGE_CURVE ( 'NONE', #18184, #4076, #29477, .T. ) ;
#24948=EDGE_CURVE ( 'NONE', #3951, #28893, #6989, .T. ) ;
#24961=CIRCLE ( 'NONE', #10296, 5.249999999999991118 ) ;
#25002=CIRCLE ( 'NONE', #27165, 24.99999999999999289 ) ;
#25008=DIRECTION ( 'NONE',  ( -0.000000000000000000, -0.000000000000000000, 1.000000000000000000 ) ) ;
#25181=CARTESIAN_POINT ( 'NONE',  ( -125.0000000000000000, 0.000000000000000000, 20.00000000000000000 ) ) ;
#25182=DIRECTION ( 'NONE',  ( 1.000000000000000000, 0.000000000000000000, 0.000000000000000000 ) ) ;
#25215=AXIS2_PLACEMENT_3D ( 'NONE', #33250, #4971, #33423 ) ;
#25220=( NAMED_UNIT ( * ) SI_UNIT ( $, .STERADIAN. ) SOLID_ANGLE_UNIT ( ) );
#25241=ORIENTED_EDGE ( 'NONE', *, *, #29511, .F. ) ;
#25305=DIRECTION ( 'NONE',  ( 1.000000000000000000, 1.804112415015879625E-16, 0.000000000000000000 ) ) ;
#25336=DIRECTION ( 'NONE',  ( -0.000000000000000000, -0.000000000000000000, 1.000000000000000000 ) ) ;
#25341=CARTESIAN_POINT ( 'NONE',  ( 125.0000000000000000, 4.592425496802574367E-14, -35.00000000000000000 ) ) ;
#25342=EDGE_CURVE ( 'NONE', #6856, #27493, #20943, .T. ) ;
#25353=CARTESIAN_POINT ( 'NONE',  ( 125.0000000000000000, 25.00000000000004619, 35.00000000000000000 ) ) ;
#25391=EDGE_CURVE ( 'NONE', #10405, #23340, #2646, .T. ) ;
#25415=AXIS2_PLACEMENT_3D ( 'NONE', #8871, #18773, #16041 ) ;
#25420=ORIENTED_EDGE ( 'NONE', *, *, #18979, .F. ) ;
#25425=EDGE_LOOP ( 'NONE', ( #19770, #9670 ) ) ;
#25448=CARTESIAN_POINT ( 'NONE',  ( -125.0000000000000000, -25.00000000000000000, -35.00000000000000000 ) ) ;
#25453=ORIENTED_EDGE ( 'NONE', *, *, #20177, .T. ) ;
#25480=CARTESIAN_POINT ( 'NONE',  ( -128.2263702798683767, 4.198250922590450074, 35.00001200000001234 ) ) ;
#25526=CARTESIAN_POINT ( 'NONE',  ( -125.0000000000000000, 25.00000000000000000, -35.00000000000000000 ) ) ;
#25533=CARTESIAN_POINT ( 'NONE',  ( -130.2500000000000000, 6.429395695523609083E-16, 35.00000599999999906 ) ) ;
#25548=ORIENTED_EDGE ( 'NONE', *, *, #3126, .F. ) ;
#25646=CIRCLE ( 'NONE', #3309, 19.99999999999998934 ) ;
#25652=CARTESIAN_POINT ( 'NONE',  ( -120.4126214611401338, 2.643999646947222892, 35.00001199999999812 ) ) ;
#25696=DIRECTION ( 'NONE',  ( -1.000000000000000000, -1.804112415015879378E-16, 0.000000000000000000 ) ) ;
#25704=ORIENTED_EDGE ( 'NONE', *, *, #6446, .T. ) ;
#25767=ORIENTED_EDGE ( 'NONE', *, *, #28341, .T. ) ;
#25810=CIRCLE ( 'NONE', #30155, 19.99999999999998934 ) ;
#25834=ADVANCED_FACE ( 'NONE', ( #10527, #9844, #7796, #4560, #10022 ), #22953, .T. ) ;
#25857=ORIENTED_EDGE ( 'NONE', *, *, #25342, .F. ) ;
#25868=FACE_OUTER_BOUND ( 'NONE', #8821, .T. ) ;
#25875=B_SPLINE_CURVE_WITH_KNOTS ( 'NONE', 3,
 ( #5154, #15542, #9935, #18440, #20490, #2101, #218, #10615, #12488, #53, #7720, #30722, #31226, #30893, #15377, #7382, #17944, #17761 ),
 .UNSPECIFIED., .F., .F.,
 ( 4, 2, 2, 2, 2, 2, 2, 2, 4 ),
 ( 0.000000000000000000, 0.06250000000000059674, 0.1250000000000012212, 0.1875000000000018874, 0.2500000000000024980, 0.3125000000000018874, 0.3750000000000012212, 0.4375000000000006106, 0.5000000000000000000 ),
 .UNSPECIFIED. ) ;
#25885=ORIENTED_EDGE ( 'NONE', *, *, #25391, .F. ) ;
#25917=LINE ( 'NONE', #18255, #28965 ) ;
#25952=DIRECTION ( 'NONE',  ( -0.000000000000000000, -0.000000000000000000, 1.000000000000000000 ) ) ;
#25989=EDGE_CURVE ( 'NONE', #28893, #33143, #15155, .T. ) ;
#26042=FACE_OUTER_BOUND ( 'NONE', #9533, .T. ) ;
#26065=EDGE_CURVE ( 'NONE', #16785, #3951, #22228, .T. ) ;
#26075=SURFACE_STYLE_FILL_AREA ( #33569 ) ;
#26121=CARTESIAN_POINT ( 'NONE',  ( -125.0000000000000000, -25.00000000000000000, 35.00000000000000000 ) ) ;
#26143=ORIENTED_EDGE ( 'NONE', *, *, #7663, .T. ) ;
#26185=DIRECTION ( 'NONE',  ( -0.000000000000000000, -0.000000000000000000, 1.000000000000000000 ) ) ;
#26301=ORIENTED_EDGE ( 'NONE', *, *, #29585, .T. ) ;
#26308=STYLED_ITEM ( 'NONE', ( #12612 ), #11883 ) ;
#26379=ORIENTED_EDGE ( 'NONE', *, *, #20375, .F. ) ;
#26458=ORIENTED_EDGE ( 'NONE', *, *, #2027, .F. ) ;
#26473=EDGE_CURVE ( 'NONE', #3669, #6381, #27581, .T. ) ;
#26552=EDGE_CURVE ( 'NONE', #33143, #1032, #8548, .T. ) ;
#26570=ORIENTED_EDGE ( 'NONE', *, *, #5485, .T. ) ;
#26578=AXIS2_PLACEMENT_3D ( 'NONE', #7763, #17808, #25305 ) ;
#26604=CARTESIAN_POINT ( 'NONE',  ( -150.0000000000000000, 0.000000000000000000, 35.00000000000000000 ) ) ;
#26613=DIRECTION ( 'NONE',  ( 0.000000000000000000, 0.000000000000000000, 1.000000000000000000 ) ) ;
#26788=VECTOR ( 'NONE', #8606, 1000.000000000000000 ) ;
#26885=VECTOR ( 'NONE', #3212, 1000.000000000000000 ) ;
#26989=EDGE_CURVE ( 'NONE', #12552, #16947, #6916, .T. ) ;
#26990=ORIENTED_EDGE ( 'NONE', *, *, #30439, .F. ) ;
#26993=CLOSED_SHELL ( 'NONE', ( #32289, #27292, #2846, #29299, #29542, #8156, #22475, #6896, #10726, #10610, #25834, #15860, #24162, #791, #1793, #14782, #12902, #3542, #15781, #9293, #10398, #13132, #30641, #11666, #21329, #24779, #20764, #13130, #14872, #20355 ) ) ;
#27066=AXIS2_PLACEMENT_3D ( 'NONE', #5759, #16152, #5928 ) ;
#27091=CIRCLE ( 'NONE', #12977, 5.249999999999991118 ) ;
#27151=DIRECTION ( 'NONE',  ( 0.000000000000000000, 0.000000000000000000, 1.000000000000000000 ) ) ;
#27165=AXIS2_PLACEMENT_3D ( 'NONE', #3275, #16059, #5996 ) ;
#27195=CARTESIAN_POINT ( 'NONE',  ( 125.6872233929728395, -5.249999999999975131, 35.00001200000001234 ) ) ;
#27225=EDGE_LOOP ( 'NONE', ( #31426, #24153 ) ) ;
#27236=PLANE ( 'NONE',  #32870 ) ;
#27248=ORIENTED_EDGE ( 'NONE', *, *, #27992, .F. ) ;
#27268=AXIS2_PLACEMENT_3D ( 'NONE', #28070, #16999, #9504 ) ;
#27269=SURFACE_SIDE_STYLE ('',( #9378 ) ) ;
#27270=DIRECTION ( 'NONE',  ( 0.000000000000000000, 0.000000000000000000, -1.000000000000000000 ) ) ;
#27292=ADVANCED_FACE ( 'NONE', ( #7937 ), #2819, .F. ) ;
#27318=CARTESIAN_POINT ( 'NONE',  ( -150.0000000000000000, 0.000000000000000000, -20.00000000000000000 ) ) ;
#27362=FACE_OUTER_BOUND ( 'NONE', #449, .T. ) ;
#27386=LINE ( 'NONE', #19559, #23789 ) ;
#27403=DIRECTION ( 'NONE',  ( -0.000000000000000000, -0.000000000000000000, 1.000000000000000000 ) ) ;
#27462=ORIENTED_EDGE ( 'NONE', *, *, #23076, .T. ) ;
#27482=FACE_BOUND ( 'NONE', #25425, .T. ) ;
#27493=VERTEX_POINT ( 'NONE', #27318 ) ;
#27548=CARTESIAN_POINT ( 'NONE',  ( 60.00000000000000000, 7.347880794884118356E-15, 35.00000000000000000 ) ) ;
#27581=CIRCLE ( 'NONE', #10721, 19.99999999999998934 ) ;
#27625=VECTOR ( 'NONE', #24804, 1000.000000000000000 ) ;
#27697=DIRECTION ( 'NONE',  ( -0.000000000000000000, -0.000000000000000000, -1.000000000000000000 ) ) ;
#27730=ORIENTED_EDGE ( 'NONE', *, *, #7663, .F. ) ;
#27756=VECTOR ( 'NONE', #676, 1000.000000000000000 ) ;
#27757=ORIENTED_EDGE ( 'NONE', *, *, #12425, .F. ) ;
#27759=VERTEX_POINT ( 'NONE', #1937 ) ;
#27863=CARTESIAN_POINT ( 'NONE',  ( -119.7499999999999858, -0.6872233929727689095, 35.00001199999999812 ) ) ;
#27974=ORIENTED_EDGE ( 'NONE', *, *, #26552, .T. ) ;
#27992=EDGE_CURVE ( 'NONE', #31209, #1032, #29004, .T. ) ;
#28036=CARTESIAN_POINT ( 'NONE',  ( -119.8866434474913660, 1.374176392886222065, 35.00001199999999812 ) ) ;
#28045=EDGE_CURVE ( 'NONE', #8245, #17833, #16713, .T. ) ;
#28070=CARTESIAN_POINT ( 'NONE',  ( -60.00000000000000000, -7.347880794884118356E-15, -20.00000000000000355 ) ) ;
#28082=EDGE_CURVE ( 'NONE', #22384, #10127, #20003, .T. ) ;
#28146=CIRCLE ( 'NONE', #25415, 24.99999999999999289 ) ;
#28244=CARTESIAN_POINT ( 'NONE',  ( -125.0000000000000000, -25.00000000000000000, 20.00000000000000000 ) ) ;
#28248=ORIENTED_EDGE ( 'NONE', *, *, #31855, .F. ) ;
#28341=EDGE_CURVE ( 'NONE', #3832, #20128, #20027, .T. ) ;
#28348=EDGE_CURVE ( 'NONE', #13595, #20519, #17058, .T. ) ;
#28462=EDGE_CURVE ( 'NONE', #10127, #22384, #30369, .T. ) ;
#28508=PRODUCT ( 'Heavy-Duty Caliper Body Housing', 'Heavy-Duty Caliper Body Housing', '', ( #8831 ) ) ;
#28527=DIRECTION ( 'NONE',  ( -1.000000000000000000, 0.000000000000000000, 0.000000000000000000 ) ) ;
#28540=AXIS2_PLACEMENT_3D ( 'NONE', #27548, #25336, #7118 ) ;
#28640=DIRECTION ( 'NONE',  ( -0.000000000000000000, -0.000000000000000000, -1.000000000000000000 ) ) ;
#28647=ORIENTED_EDGE ( 'NONE', *, *, #1818, .F. ) ;
#28744=EDGE_CURVE ( 'NONE', #12431, #7668, #29635, .T. ) ;
#28774=DIRECTION ( 'NONE',  ( -0.000000000000000000, -0.000000000000000000, 1.000000000000000000 ) ) ;
#28878=AXIS2_PLACEMENT_3D ( 'NONE', #4570, #4055, #1340 ) ;
#28893=VERTEX_POINT ( 'NONE', #16675 ) ;
#28936=ORIENTED_EDGE ( 'NONE', *, *, #3089, .F. ) ;
#28938=EDGE_CURVE ( 'NONE', #20128, #32783, #2025, .T. ) ;
#28941=DIRECTION ( 'NONE',  ( -0.000000000000000000, -0.000000000000000000, 1.000000000000000000 ) ) ;
#28965=VECTOR ( 'NONE', #2080, 1000.000000000000000 ) ;
#29004=LINE ( 'NONE', #26121, #15654 ) ;
#29015=CIRCLE ( 'NONE', #182, 5.250000000000004441 ) ;
#29085=FACE_OUTER_BOUND ( 'NONE', #16607, .T. ) ;
#29110=CYLINDRICAL_SURFACE ( 'NONE', #27066, 24.99999999999999289 ) ;
#29140=CARTESIAN_POINT ( 'NONE',  ( 125.0000000000000000, -24.99999999999995737, 20.00000000000000000 ) ) ;
#29166=LINE ( 'NONE', #26604, #13271 ) ;
#29248=FACE_BOUND ( 'NONE', #8338, .T. ) ;
#29250=CARTESIAN_POINT ( 'NONE',  ( 129.5873785388598947, -2.643999646947195359, 35.00001200000000523 ) ) ;
#29256=EDGE_CURVE ( 'NONE', #23340, #12431, #30995, .T. ) ;
#29267=ORIENTED_EDGE ( 'NONE', *, *, #28082, .F. ) ;
#29299=ADVANCED_FACE ( 'NONE', ( #26042 ), #2367, .F. ) ;
#29328=DIRECTION ( 'NONE',  ( -1.000000000000000000, -1.804112415015879378E-16, -0.000000000000000000 ) ) ;
#29340=DIRECTION ( 'NONE',  ( -0.000000000000000000, -0.000000000000000000, -1.000000000000000000 ) ) ;
#29351=CARTESIAN_POINT ( 'NONE',  ( -125.0000000000000000, 0.000000000000000000, 35.00000000000000000 ) ) ;
#29403=ORIENTED_EDGE ( 'NONE', *, *, #11473, .T. ) ;
#29413=CYLINDRICAL_SURFACE ( 'NONE', #9927, 5.249999999999991118 ) ;
#29477=LINE ( 'NONE', #5644, #20019 ) ;
#29511=EDGE_CURVE ( 'NONE', #32783, #21298, #8839, .T. ) ;
#29523=PRODUCT_DEFINITION_CONTEXT ( 'detailed design', #24200, 'design' ) ;
#29542=ADVANCED_FACE ( 'NONE', ( #27362 ), #22590, .F. ) ;
#29573=EDGE_LOOP ( 'NONE', ( #16316, #18670, #451, #33549 ) ) ;
#29585=EDGE_CURVE ( 'NONE', #2221, #29773, #31491, .T. ) ;
#29612=VERTEX_POINT ( 'NONE', #14586 ) ;
#29635=LINE ( 'NONE', #23846, #22187 ) ;
#29638=CARTESIAN_POINT ( 'NONE',  ( -60.00000000000000000, -7.347880794884118356E-15, 35.00000000000000000 ) ) ;
#29651=ORIENTED_EDGE ( 'NONE', *, *, #5182, .F. ) ;
#29773=VERTEX_POINT ( 'NONE', #10507 ) ;
#29788=CARTESIAN_POINT ( 'NONE',  ( 60.00000000000000000, 7.347880794884118356E-15, 35.00000000000000000 ) ) ;
#29801=DIRECTION ( 'NONE',  ( 0.000000000000000000, 0.000000000000000000, 1.000000000000000000 ) ) ;
#29820=CIRCLE ( 'NONE', #12403, 24.99999999999999289 ) ;
#29837=CARTESIAN_POINT ( 'NONE',  ( -60.00000000000000000, -7.347880794884118356E-15, -20.00000000000000355 ) ) ;
#29845=CARTESIAN_POINT ( 'NONE',  ( 130.2499999999999716, 2.997323040913146538E-14, 35.00000599999999906 ) ) ;
#29848=DIRECTION ( 'NONE',  ( 1.000000000000000000, 0.000000000000000000, 0.000000000000000000 ) ) ;
#29957=CARTESIAN_POINT ( 'NONE',  ( -125.0000000000000000, -25.00000000000000000, 35.00000000000000000 ) ) ;
#29966=DIRECTION ( 'NONE',  ( 0.000000000000000000, 0.000000000000000000, 1.000000000000000000 ) ) ;
#30029=EDGE_LOOP ( 'NONE', ( #6389, #11963, #17159, #28647, #17328 ) ) ;
#30155=AXIS2_PLACEMENT_3D ( 'NONE', #21766, #8816, #23825 ) ;
#30168=( NAMED_UNIT ( * ) SI_UNIT ( $, .STERADIAN. ) SOLID_ANGLE_UNIT ( ) );
#30181=CARTESIAN_POINT ( 'NONE',  ( -125.0000000000000000, 0.000000000000000000, -35.00000000000000000 ) ) ;
#30186=CARTESIAN_POINT ( 'NONE',  ( -65.24999999999998579, -6.704941225331758828E-15, -35.00000000000000000 ) ) ;
#30261=DIRECTION ( 'NONE',  ( 1.000000000000000000, 0.000000000000000000, 0.000000000000000000 ) ) ;
#30312=ORIENTED_EDGE ( 'NONE', *, *, #11183, .T. ) ;
#30334=PRESENTATION_STYLE_ASSIGNMENT (( #22154 ) ) ;
#30369=CIRCLE ( 'NONE', #9691, 5.250000000000004441 ) ;
#30370=CARTESIAN_POINT ( 'NONE',  ( -60.00000000000000000, -7.347880794884118356E-15, 20.00000000000000000 ) ) ;
#30419=EDGE_CURVE ( 'NONE', #18729, #2221, #5467, .T. ) ;
#30437=CARTESIAN_POINT ( 'NONE',  ( -124.3127766070272315, -5.250000000000003553, 35.00001199999999812 ) ) ;
#30439=EDGE_CURVE ( 'NONE', #20133, #28893, #5296, .T. ) ;
#30484=EDGE_LOOP ( 'NONE', ( #10352, #15406, #4842, #11299 ) ) ;
#30490=ORIENTED_EDGE ( 'NONE', *, *, #9346, .F. ) ;
#30535=CIRCLE ( 'NONE', #3868, 5.249999999999997335 ) ;
#30600=CARTESIAN_POINT ( 'NONE',  ( -126.3741763928861985, 5.113356552508657948, 35.00001199999999812 ) ) ;
#30637=CARTESIAN_POINT ( 'NONE',  ( 125.0000000000000000, 3.061616997868383121E-14, -20.00000000000000355 ) ) ;
#30641=ADVANCED_FACE ( 'NONE', ( #4315, #27482, #20151, #11813, #17098 ), #6870, .F. ) ;
#30690=STYLED_ITEM ( 'NONE', ( #30334 ), #31568 ) ;
#30712=ORIENTED_EDGE ( 'NONE', *, *, #3126, .T. ) ;
#30722=CARTESIAN_POINT ( 'NONE',  ( 122.3560003530527638, 4.587378538859887556, 35.00001199999999812 ) ) ;
#30836=EDGE_LOOP ( 'NONE', ( #31126, #21446 ) ) ;
#30841=EDGE_LOOP ( 'NONE', ( #23161, #9878, #29403, #998 ) ) ;
#30893=CARTESIAN_POINT ( 'NONE',  ( 120.8017490774095251, 3.226370279868335800, 35.00001199999999102 ) ) ;
#30967=ORIENTED_EDGE ( 'NONE', *, *, #24920, .T. ) ;
#30971=EDGE_CURVE ( 'NONE', #6381, #3669, #7594, .T. ) ;
#30974=DIRECTION ( 'NONE',  ( 1.000000000000000000, 0.000000000000000000, 0.000000000000000000 ) ) ;
#30995=LINE ( 'NONE', #10209, #12442 ) ;
#31015=CARTESIAN_POINT ( 'NONE',  ( -119.7500000000000000, 0.000000000000000000, -35.00000000000000000 ) ) ;
#31068=CARTESIAN_POINT ( 'NONE',  ( -65.25000000000000000, -6.704941225331758039E-15, 35.00000000000000000 ) ) ;
#31080=CARTESIAN_POINT ( 'NONE',  ( 65.25000000000000000, 7.347880794884118356E-15, 35.00000000000000000 ) ) ;
#31126=ORIENTED_EDGE ( 'NONE', *, *, #31198, .T. ) ;
#31146=CARTESIAN_POINT ( 'NONE',  ( -105.0000000000000142, 2.449293598294705330E-15, 20.00000000000000000 ) ) ;
#31198=EDGE_CURVE ( 'NONE', #17833, #8245, #2555, .T. ) ;
#31209=VERTEX_POINT ( 'NONE', #29957 ) ;
#31215=ORIENTED_EDGE ( 'NONE', *, *, #14305, .F. ) ;
#31217=CIRCLE ( 'NONE', #25215, 5.249999999999991118 ) ;
#31226=CARTESIAN_POINT ( 'NONE',  ( 121.7736297201317370, 4.198250922590482048, 35.00001200000001234 ) ) ;
#31244=EDGE_LOOP ( 'NONE', ( #6733, #5714 ) ) ;
#31256=EDGE_CURVE ( 'NONE', #18960, #4076, #31372, .T. ) ;
#31308=DIRECTION ( 'NONE',  ( -0.000000000000000000, -0.000000000000000000, -1.000000000000000000 ) ) ;
#31336=DIRECTION ( 'NONE',  ( -0.000000000000000000, -0.000000000000000000, 1.000000000000000000 ) ) ;
#31372=CIRCLE ( 'NONE', #4165, 5.249999999999997335 ) ;
#31375=ORIENTED_EDGE ( 'NONE', *, *, #18979, .T. ) ;
#31404=ORIENTED_EDGE ( 'NONE', *, *, #5404, .T. ) ;
#31426=ORIENTED_EDGE ( 'NONE', *, *, #2946, .F. ) ;
#31460=ORIENTED_EDGE ( 'NONE', *, *, #24920, .F. ) ;
#31464=ORIENTED_EDGE ( 'NONE', *, *, #17275, .F. ) ;
#31484=CARTESIAN_POINT ( 'NONE',  ( 120.8017490774095535, -3.226370279868274515, 35.00001200000000523 ) ) ;
#31491=CIRCLE ( 'NONE', #14601, 19.99999999999998934 ) ;
#31568=ADVANCED_BREP_SHAPE_REPRESENTATION ( '', ( #11883, #2404 ), #33408 ) ;
#31703=ORIENTED_EDGE ( 'NONE', *, *, #8088, .T. ) ;
#31710=ORIENTED_EDGE ( 'NONE', *, *, #28045, .F. ) ;
#31825=FACE_OUTER_BOUND ( 'NONE', #8283, .T. ) ;
#31831=DIRECTION ( 'NONE',  ( -0.000000000000000000, -0.000000000000000000, 1.000000000000000000 ) ) ;
#31855=EDGE_CURVE ( 'NONE', #5501, #29612, #5409, .T. ) ;
#31862=ORIENTED_EDGE ( 'NONE', *, *, #20533, .T. ) ;
#31863=DIRECTION ( 'NONE',  ( 1.000000000000000000, 0.000000000000000000, 0.000000000000000000 ) ) ;
#31903=AXIS2_PLACEMENT_3D ( 'NONE', #12297, #9239, #17073 ) ;
#31936=LINE ( 'NONE', #3322, #26788 ) ;
#31942=ORIENTED_EDGE ( 'NONE', *, *, #29511, .T. ) ;
#31955=AXIS2_PLACEMENT_3D ( 'NONE', #3781, #24561, #21499 ) ;
#31989=DIRECTION ( 'NONE',  ( -0.000000000000000000, -0.000000000000000000, 1.000000000000000000 ) ) ;
#32032=AXIS2_PLACEMENT_3D ( 'NONE', #709, #1048, #19270 ) ;
#32066=ORIENTED_EDGE ( 'NONE', *, *, #23461, .T. ) ;
#32131=PLANE ( 'NONE',  #17531 ) ;
#32289=ADVANCED_FACE ( 'NONE', ( #19243 ), #8198, .F. ) ;
#32346=DIRECTION ( 'NONE',  ( 1.000000000000000000, 0.000000000000000000, -0.000000000000000000 ) ) ;
#32399=ORIENTED_EDGE ( 'NONE', *, *, #28744, .F. ) ;
#32406=EDGE_LOOP ( 'NONE', ( #4294, #20939, #31942, #19639 ) ) ;
#32452=DIRECTION ( 'NONE',  ( 0.000000000000000000, 0.000000000000000000, 1.000000000000000000 ) ) ;
#32470=CARTESIAN_POINT ( 'NONE',  ( -120.8017490774095535, -3.226370279868306046, 35.00001200000000523 ) ) ;
#32492=FACE_OUTER_BOUND ( 'NONE', #23063, .T. ) ;
#32512=DIRECTION ( 'NONE',  ( 0.000000000000000000, 0.000000000000000000, 1.000000000000000000 ) ) ;
#32528=AXIS2_PLACEMENT_3D ( 'NONE', #1850, #32512, #6968 ) ;
#32542=( NAMED_UNIT ( * ) PLANE_ANGLE_UNIT ( ) SI_UNIT ( $, .RADIAN. ) );
#32559=VECTOR ( 'NONE', #10232, 1000.000000000000000 ) ;
#32562=CARTESIAN_POINT ( 'NONE',  ( -125.0000000000000000, 0.000000000000000000, -35.00000000000000000 ) ) ;
#32642=CARTESIAN_POINT ( 'NONE',  ( -121.7736297201316660, -4.198250922590450074, 35.00001199999999102 ) ) ;
#32701=CARTESIAN_POINT ( 'NONE',  ( -130.2500000000000000, 6.429395695523608097E-16, -35.00000000000000000 ) ) ;
#32723=DIRECTION ( 'NONE',  ( -0.000000000000000000, -0.000000000000000000, 1.000000000000000000 ) ) ;
#32731=ORIENTED_EDGE ( 'NONE', *, *, #22897, .F. ) ;
#32768=VECTOR ( 'NONE', #29328, 1000.000000000000000 ) ;
#32783=VERTEX_POINT ( 'NONE', #25533 ) ;
#32808=CARTESIAN_POINT ( 'NONE',  ( -120.4126214611401480, -2.643999646947226889, 35.00001199999999812 ) ) ;
#32820=CIRCLE ( 'NONE', #2900, 5.249999999999991118 ) ;
#32870=AXIS2_PLACEMENT_3D ( 'NONE', #25181, #29966, #32346 ) ;
#32913=VERTEX_POINT ( 'NONE', #4585 ) ;
#32917=DIRECTION ( 'NONE',  ( 1.000000000000000000, 0.000000000000000000, 0.000000000000000000 ) ) ;
#33013=CARTESIAN_POINT ( 'NONE',  ( -54.75000000000000711, -7.347880794884118356E-15, 35.00000000000000000 ) ) ;
#33132=CIRCLE ( 'NONE', #32032, 24.99999999999999289 ) ;
#33143=VERTEX_POINT ( 'NONE', #7255 ) ;
#33155=CARTESIAN_POINT ( 'NONE',  ( -150.0000000000000000, 0.000000000000000000, -35.00000000000000000 ) ) ;
#33156=CARTESIAN_POINT ( 'NONE',  ( -123.6258236071138015, 5.113356552508662389, 35.00001200000000523 ) ) ;
#33196=DIRECTION ( 'NONE',  ( 1.000000000000000000, 0.000000000000000000, 0.000000000000000000 ) ) ;
#33232=FACE_OUTER_BOUND ( 'NONE', #18678, .T. ) ;
#33250=CARTESIAN_POINT ( 'NONE',  ( 60.00000000000000000, 7.347880794884118356E-15, -35.00000000000000000 ) ) ;
#33274=DIRECTION ( 'NONE',  ( -0.000000000000000000, -0.000000000000000000, 1.000000000000000000 ) ) ;
#33285=EDGE_LOOP ( 'NONE', ( #12666, #19630, #12351, #13545 ) ) ;
#33351=DIRECTION ( 'NONE',  ( 1.000000000000000000, 0.000000000000000000, 0.000000000000000000 ) ) ;
#33357=AXIS2_PLACEMENT_3D ( 'NONE', #29638, #10751, #23850 ) ;
#33384=CARTESIAN_POINT ( 'NONE',  ( 125.0000000000000000, 25.00000000000004619, -35.00000000000000000 ) ) ;
#33393=( GEOMETRIC_REPRESENTATION_CONTEXT ( 3 ) GLOBAL_UNCERTAINTY_ASSIGNED_CONTEXT ( ( #13720 ) ) GLOBAL_UNIT_ASSIGNED_CONTEXT ( ( #17903, #334, #10078 ) ) REPRESENTATION_CONTEXT ( 'NONE', 'WORKASPACE' ) );
#33408=( GEOMETRIC_REPRESENTATION_CONTEXT ( 3 ) GLOBAL_UNCERTAINTY_ASSIGNED_CONTEXT ( ( #21231 ) ) GLOBAL_UNIT_ASSIGNED_CONTEXT ( ( #6018, #24883, #25220 ) ) REPRESENTATION_CONTEXT ( 'NONE', 'WORKASPACE' ) );
#33423=DIRECTION ( 'NONE',  ( 1.000000000000000000, 0.000000000000000000, 0.000000000000000000 ) ) ;
#33521=CARTESIAN_POINT ( 'NONE',  ( -125.0000000000000000, 0.000000000000000000, 35.00000000000000000 ) ) ;
#33549=ORIENTED_EDGE ( 'NONE', *, *, #30419, .F. ) ;
#33558=ORIENTED_EDGE ( 'NONE', *, *, #23461, .F. ) ;
#33569=FILL_AREA_STYLE ('',( #16004 ) ) ;
#33627=LINE ( 'NONE', #25448, #10314 ) ;
#33681=EDGE_LOOP ( 'NONE', ( #23930, #19472, #25453, #21979 ) ) ;
ENDSEC;
END-ISO-10303-21;
